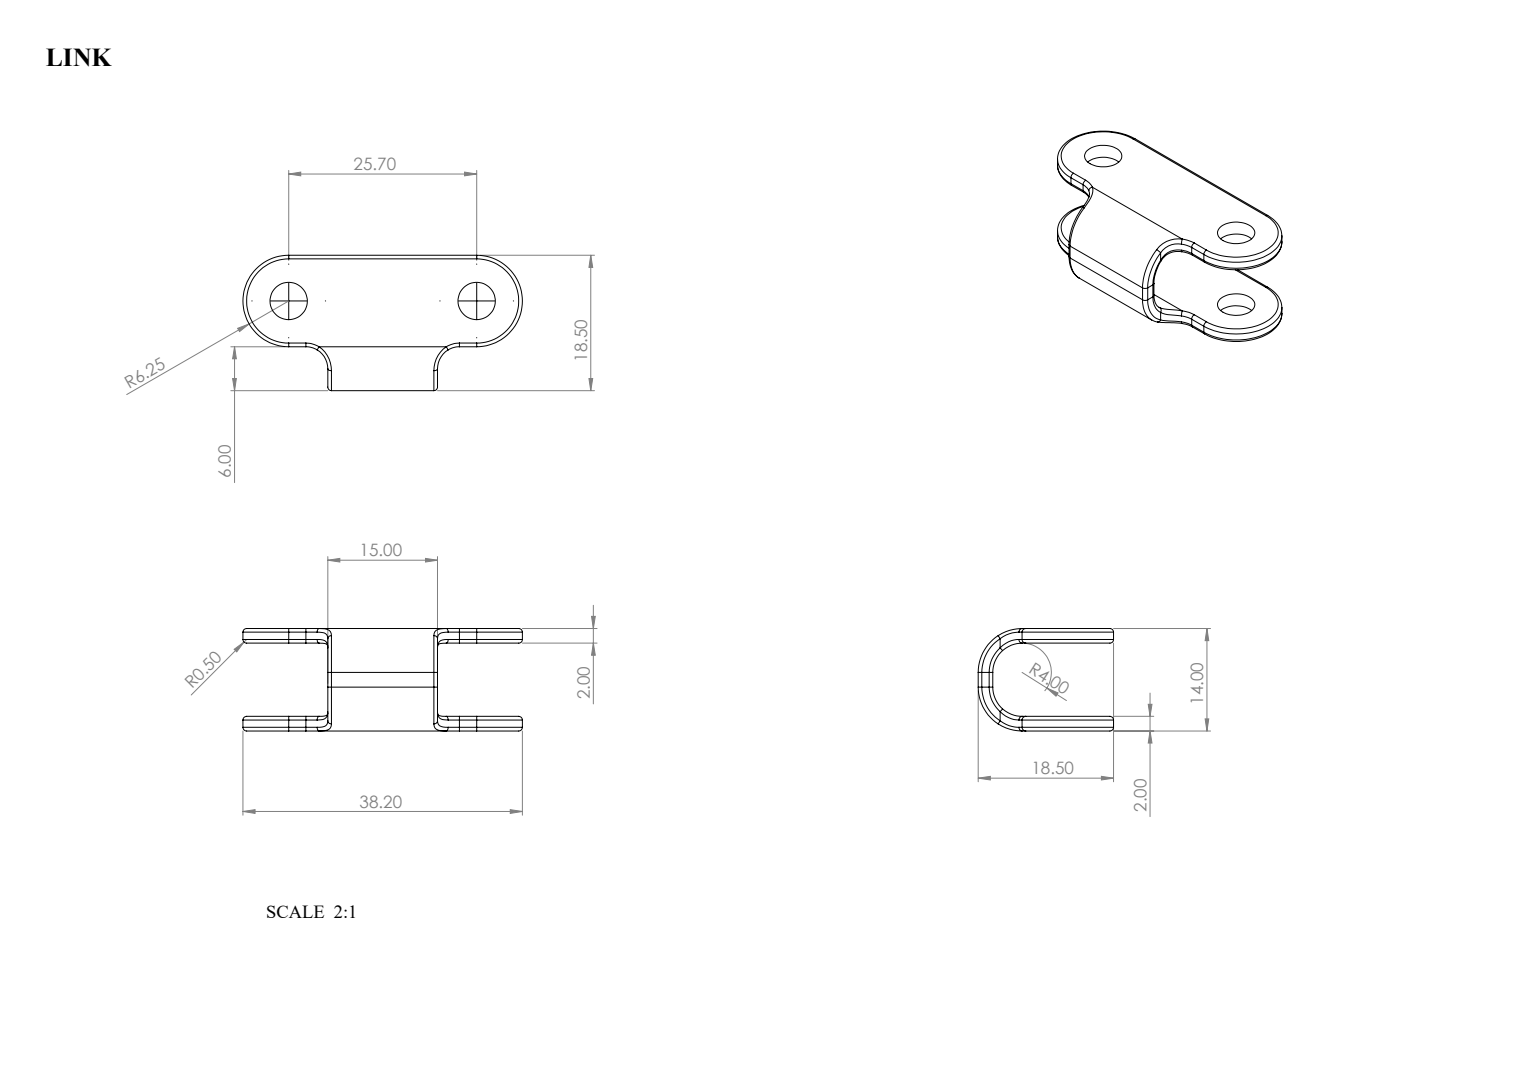
ISO-10303-21;
HEADER;
FILE_DESCRIPTION (('STEP AP214'),
    '1' );
FILE_NAME ('Link.step',
    '2026-10-06T08:09:25',
    ( '' ),
    ( '' ),
    'SwSTEP 2.0',
    'SolidWorks 2021',
    '' );
FILE_SCHEMA (( 'AUTOMOTIVE_DESIGN' ));
ENDSEC;

DATA;
#21=CARTESIAN_POINT ( 'NONE',  ( 8.498922697886333921, -1.509195795641886439, 6.997949321565420711 ) ) ;
#31=EDGE_LOOP ( 'NONE', ( #17480, #19110, #8752, #782 ) ) ;
#37=DIRECTION ( 'NONE',  ( 1.000000000000000000, 4.252453317207022018E-31, -5.551115123125818447E-17 ) ) ;
#38=ADVANCED_FACE ( 'NONE', ( #17307 ), #9922, .T. ) ;
#39=CARTESIAN_POINT ( 'NONE',  ( 7.263517083688578069, -11.72058614530574694, 7.724990489865656507 ) ) ;
#41=CARTESIAN_POINT ( 'NONE',  ( -6.999999999999978684, -10.98142396999974046, 8.916666666666724694 ) ) ;
#43=CARTESIAN_POINT ( 'NONE',  ( 7.909386411297032460, -13.36290293203342650, 7.731447622712527057 ) ) ;
#47=CARTESIAN_POINT ( 'NONE',  ( 12.84999999999997300, -1.999999999999998224, -2.550000000000000711 ) ) ;
#48=DIRECTION ( 'NONE',  ( -2.168404344971017743E-16, -1.000000000000000000, 6.982962677686261977E-15 ) ) ;
#49=DIRECTION ( 'NONE',  ( 0.000000000000000000, 0.000000000000000000, 1.000000000000000000 ) ) ;
#50=EDGE_CURVE ( 'NONE', #20148, #6938, #11790, .T. ) ;
#51=CYLINDRICAL_SURFACE ( 'NONE', #1797, 0.4999999999999995559 ) ;
#56=EDGE_LOOP ( 'NONE', ( #13558, #11700, #20158, #8031 ) ) ;
#82=CYLINDRICAL_SURFACE ( 'NONE', #15543, 0.4999999999999995559 ) ;
#89=ORIENTED_EDGE ( 'NONE', *, *, #7270, .T. ) ;
#94=CARTESIAN_POINT ( 'NONE',  ( 7.499999999999978684, 1.734723475976807094E-14, 9.249999999999980460 ) ) ;
#111=ORIENTED_EDGE ( 'NONE', *, *, #7820, .T. ) ;
#112=ORIENTED_EDGE ( 'NONE', *, *, #14818, .T. ) ;
#127=CARTESIAN_POINT ( 'NONE',  ( 7.499999999999978684, -2.645898033750298417, 9.250000000000021316 ) ) ;
#129=CARTESIAN_POINT ( 'NONE',  ( 8.697224362268009656, -1.999999999999984013, 6.249999999999998224 ) ) ;
#138=VERTEX_POINT ( 'NONE', #8274 ) ;
#149=CARTESIAN_POINT ( 'NONE',  ( 7.554637128289398262, -0.1201405311246625390, 7.453047528892632556 ) ) ;
#150=CARTESIAN_POINT ( 'NONE',  ( 8.723547172042144027, -11.98401194435536432, 6.817515300135809753 ) ) ;
#153=CARTESIAN_POINT ( 'NONE',  ( 7.000000000000006217, -11.35410196624971491, 9.250000000000008882 ) ) ;
#161=CARTESIAN_POINT ( 'NONE',  ( -12.85000000000004228, -0.5000000000000004441, -6.249999999999977796 ) ) ;
#164=DIRECTION ( 'NONE',  ( -9.121204216617949000E-31, -1.000000000000000000, 6.982962677686261977E-15 ) ) ;
#167=CARTESIAN_POINT ( 'NONE',  ( 8.204963667274160599, -0.08625821904936173401, 7.312308861538857840 ) ) ;
#193=CARTESIAN_POINT ( 'NONE',  ( -12.84999999999999964, -1.500000000000001332, 5.750000000000005329 ) ) ;
#195=VERTEX_POINT ( 'NONE', #8969 ) ;
#207=ADVANCED_FACE ( 'NONE', ( #3092, #23213, #8851 ), #10257, .T. ) ;
#208=EDGE_CURVE ( 'NONE', #21919, #22681, #22973, .T. ) ;
#211=DIRECTION ( 'NONE',  ( 1.454462294001240516E-30, 1.000000000000000000, 0.000000000000000000 ) ) ;
#213=DIRECTION ( 'NONE',  ( -2.168404344971017743E-16, -1.000000000000000000, 6.982962677686261977E-15 ) ) ;
#215=CARTESIAN_POINT ( 'NONE',  ( -8.195710046796538251, -2.011959044857179357, 6.570882465138005557 ) ) ;
#219=CARTESIAN_POINT ( 'NONE',  ( 10.49999999999999467, -14.00000000000000888, 9.250000000000063949 ) ) ;
#224=CARTESIAN_POINT ( 'NONE',  ( -10.49999999999999467, -1.500000000000001332, 5.750000000000005329 ) ) ;
#229=ORIENTED_EDGE ( 'NONE', *, *, #14979, .F. ) ;
#236=CIRCLE ( 'NONE', #19764, 2.999999999999995559 ) ;
#241=CARTESIAN_POINT ( 'NONE',  ( 8.510464245293309915, -13.49280278100692243, 6.988717072694059063 ) ) ;
#247=ORIENTED_EDGE ( 'NONE', *, *, #13683, .T. ) ;
#255=CARTESIAN_POINT ( 'NONE',  ( 7.000000000000001776, -10.98142396999974935, 8.916666666666673180 ) ) ;
#268=CARTESIAN_POINT ( 'NONE',  ( 8.565230440156003766, -1.999999999999984457, 6.320505311736929421 ) ) ;
#270=CARTESIAN_POINT ( 'NONE',  ( 8.429621201837189659, 1.585786587480479934E-14, 6.425428529984677617 ) ) ;
#280=VERTEX_POINT ( 'NONE', #12363 ) ;
#300=FACE_OUTER_BOUND ( 'NONE', #859, .T. ) ;
#303=EDGE_CURVE ( 'NONE', #3117, #17483, #12943, .T. ) ;
#313=ORIENTED_EDGE ( 'NONE', *, *, #17284, .F. ) ;
#331=DIRECTION ( 'NONE',  ( 9.121204216617949000E-31, 1.000000000000000000, -6.982962677686261977E-15 ) ) ;
#347=CARTESIAN_POINT ( 'NONE',  ( 7.500000000000007105, -5.999999999999981348, 12.24999999999998224 ) ) ;
#353=EDGE_CURVE ( 'NONE', #9717, #9721, #18241, .T. ) ;
#358=CARTESIAN_POINT ( 'NONE',  ( 7.651206356577058720, -13.16616768173521912, 8.300907142094251512 ) ) ;
#359=DIRECTION ( 'NONE',  ( 1.000000000000000000, 1.910522504832140594E-31, -5.551115123125818447E-17 ) ) ;
#392=CARTESIAN_POINT ( 'NONE',  ( 7.345446946324464932, -0.2181520686730648306, 7.860330092053914974 ) ) ;
#396=VERTEX_POINT ( 'NONE', #16803 ) ;
#398=ORIENTED_EDGE ( 'NONE', *, *, #14716, .T. ) ;
#403=CYLINDRICAL_SURFACE ( 'NONE', #5007, 2.549999999999997158 ) ;
#404=( BOUNDED_SURFACE ( )  B_SPLINE_SURFACE ( 3, 2, ( 
 ( #12933, #11388, #19885 ),
 ( #2337, #3867, #21995 ),
 ( #16676, #20341, #11045 ),
 ( #16449, #5881, #465 ),
 ( #1987, #21769, #358 ),
 ( #5654, #9411, #3752 ),
 ( #13050, #20237, #11166 ),
 ( #587, #6112, #14923 ),
 ( #7871, #22109, #18578 ),
 ( #6001, #16555, #7527 ),
 ( #2228, #15035, #10918 ),
 ( #9177, #16338, #241 ),
 ( #7412, #20827, #6346 ),
 ( #4690, #13397, #13518 ) ),
 .UNSPECIFIED., .F., .F., .F. ) 
 B_SPLINE_SURFACE_WITH_KNOTS ( ( 4, 2, 2, 2, 2, 2, 4 ),
 ( 3, 3 ),
 ( 0.000000000000000000, 0.0009385527998839217345, 0.001407829199825882602, 0.001877105599767843469, 0.002346381999709804336, 0.002815658399651765204, 0.003754211199535686938 ),
 ( 0.000000000000000000, 1.000000000000000000 ),
 .UNSPECIFIED. ) 
 GEOMETRIC_REPRESENTATION_ITEM ( )  RATIONAL_B_SPLINE_SURFACE ( (
 ( 1.000000000000000000, 0.7071067811865469066, 1.000000000000000000),
 ( 1.000000000000000000, 0.7217349950160889538, 1.000000000000000000),
 ( 1.000000000000000000, 0.7325631490734629825, 1.000000000000000000),
 ( 1.000000000000000000, 0.7426392126584471232, 1.000000000000000000),
 ( 1.000000000000000000, 0.7449451721693458595, 1.000000000000000000),
 ( 1.000000000000000000, 0.7474053618999159099, 1.000000000000000000),
 ( 1.000000000000000000, 0.7475947887410098192, 1.000000000000000000),
 ( 1.000000000000000000, 0.7461109904165789120, 1.000000000000000000),
 ( 1.000000000000000000, 0.7444113185333037785, 1.000000000000000000),
 ( 1.000000000000000000, 0.7395217850810181792, 1.000000000000000000),
 ( 1.000000000000000000, 0.7363545993504778675, 1.000000000000000000),
 ( 1.000000000000000000, 0.7253814056383908193, 1.000000000000000000),
 ( 1.000000000000000000, 0.7159765610437973660, 1.000000000000000000),
 ( 1.000000000000000000, 0.7071067811865494601, 1.000000000000000000) ) ) 
 REPRESENTATION_ITEM ( '' )  SURFACE ( )  );
#406=ORIENTED_EDGE ( 'NONE', *, *, #6745, .T. ) ;
#413=FACE_OUTER_BOUND ( 'NONE', #17566, .T. ) ;
#420=ORIENTED_EDGE ( 'NONE', *, *, #15029, .F. ) ;
#422=ORIENTED_EDGE ( 'NONE', *, *, #14825, .T. ) ;
#431=CARTESIAN_POINT ( 'NONE',  ( -12.85000000000001386, -14.00000000000005329, 2.550000000000052669 ) ) ;
#453=CARTESIAN_POINT ( 'NONE',  ( -12.84999999999999964, -0.5000000000000038858, 5.750000000000018652 ) ) ;
#458=AXIS2_PLACEMENT_3D ( 'NONE', #20608, #18832, #22132 ) ;
#463=AXIS2_PLACEMENT_3D ( 'NONE', #5270, #12430, #19613 ) ;
#465=CARTESIAN_POINT ( 'NONE',  ( 7.613388670473287156, -13.11165441297993084, 8.423574099071744925 ) ) ;
#469=PRESENTATION_STYLE_ASSIGNMENT (( #14587 ) ) ;
#476=CIRCLE ( 'NONE', #11356, 0.4999999999999998335 ) ;
#479=AXIS2_PLACEMENT_3D ( 'NONE', #21483, #5360, #14060 ) ;
#501=DIRECTION ( 'NONE',  ( 1.454462294001240516E-30, 1.000000000000000000, 0.000000000000000000 ) ) ;
#508=CARTESIAN_POINT ( 'NONE',  ( 7.000000000000009770, -0.9711575687493200215, 9.522727272727296466 ) ) ;
#523=CIRCLE ( 'NONE', #891, 4.000000000000000000 ) ;
#525=AXIS2_PLACEMENT_3D ( 'NONE', #3093, #22741, #3329 ) ;
#526=DIRECTION ( 'NONE',  ( -1.000000000000000000, -6.224605580259554159E-31, 2.887593071917436153E-31 ) ) ;
#532=DIRECTION ( 'NONE',  ( -1.000000000000000000, 2.312964634635739999E-16, -1.302601544865244959E-30 ) ) ;
#538=VECTOR ( 'NONE', #11676, 1000.000000000000000 ) ;
#540=ORIENTED_EDGE ( 'NONE', *, *, #22390, .T. ) ;
#562=CARTESIAN_POINT ( 'NONE',  ( -8.422565759993579704, -12.00000000000004441, 6.396710472006764903 ) ) ;
#563=CARTESIAN_POINT ( 'NONE',  ( -7.604097569491910846, -13.58924811263090504, 8.440516644273101221 ) ) ;
#579=CARTESIAN_POINT ( 'NONE',  ( -8.954763739086851970, -12.50000000000002132, 6.678571428571506097 ) ) ;
#587=CARTESIAN_POINT ( 'NONE',  ( 7.490313984279763027, -13.85571552873294365, 7.566633644154762806 ) ) ;
#597=EDGE_CURVE ( 'NONE', #11755, #7710, #15633, .T. ) ;
#605=ORIENTED_EDGE ( 'NONE', *, *, #6240, .F. ) ;
#617=EDGE_CURVE ( 'NONE', #18641, #4863, #6775, .T. ) ;
#618=FACE_OUTER_BOUND ( 'NONE', #20038, .T. ) ;
#635=VERTEX_POINT ( 'NONE', #18338 ) ;
#639=CYLINDRICAL_SURFACE ( 'NONE', #14898, 2.549999999999997158 ) ;
#642=CARTESIAN_POINT ( 'NONE',  ( 8.954763739086866181, -13.50000000000002309, 6.678571428571478563 ) ) ;
#706=CARTESIAN_POINT ( 'NONE',  ( 8.160037397871480636, -13.99120688549555425, 6.662331851012024408 ) ) ;
#711=FILL_AREA_STYLE_COLOUR ( '', #14886 ) ;
#723=ADVANCED_FACE ( 'NONE', ( #1644 ), #6821, .F. ) ;
#734=DIRECTION ( 'NONE',  ( -2.168404344970994323E-16, 1.000000000000000000, -1.577721810442023611E-30 ) ) ;
#742=ORIENTED_EDGE ( 'NONE', *, *, #2797, .T. ) ;
#760=CARTESIAN_POINT ( 'NONE',  ( -7.521298409251860662, -2.242072331701493670, 8.817899680514866390 ) ) ;
#765=CARTESIAN_POINT ( 'NONE',  ( -12.84999999999999964, -2.000000000000001776, 0.000000000000000000 ) ) ;
#780=ORIENTED_EDGE ( 'NONE', *, *, #14197, .F. ) ;
#782=ORIENTED_EDGE ( 'NONE', *, *, #10105, .F. ) ;
#791=AXIS2_PLACEMENT_3D ( 'NONE', #11762, #9654, #13189 ) ;
#793=CARTESIAN_POINT ( 'NONE',  ( -7.568091547083489523, -11.30436690654930310, 8.516664522246358615 ) ) ;
#794=CARTESIAN_POINT ( 'NONE',  ( -7.856071383949657871, -13.95231939088843021, 7.015054140272262373 ) ) ;
#799=CARTESIAN_POINT ( 'NONE',  ( -12.84999999999999964, -1.500000000000001332, 5.750000000000005329 ) ) ;
#807=CARTESIAN_POINT ( 'NONE',  ( -12.84999999999999964, -1.500000000000001332, 0.000000000000000000 ) ) ;
#809=B_SPLINE_CURVE_WITH_KNOTS ( 'NONE', 3,
 ( #13972, #21165, #12198, #1513, #14095, #21281, #3840, #18320, #5628, #11357, #21972, #19968, #19857, #9491, #4079, #7847 ),
 .UNSPECIFIED., .F., .F.,
 ( 4, 2, 2, 2, 2, 2, 2, 4 ),
 ( 2.168404344970985372E-18, 0.0008458391445145506393, 0.001268758716771827043, 0.001691678289029103664, 0.002114597861286380068, 0.002537517433543656688, 0.002960437005800932875, 0.003383356578058209496 ),
 .UNSPECIFIED. ) ;
#810=DIRECTION ( 'NONE',  ( 1.000000000000000000, 3.081487911019581306E-31, -5.551115123125761132E-17 ) ) ;
#828=ORIENTED_EDGE ( 'NONE', *, *, #7076, .T. ) ;
#840=DIRECTION ( 'NONE',  ( 1.000000000000000000, -2.168404344971017743E-16, 1.203141491611691375E-30 ) ) ;
#848=DIRECTION ( 'NONE',  ( 2.168404344971008868E-16, 1.000000000000000000, 0.000000000000000000 ) ) ;
#859=EDGE_LOOP ( 'NONE', ( #22643, #18058, #20307, #6787 ) ) ;
#877=EDGE_CURVE ( 'NONE', #9710, #18942, #14680, .T. ) ;
#891=AXIS2_PLACEMENT_3D ( 'NONE', #18596, #17276, #8120 ) ;
#898=ADVANCED_FACE ( 'NONE', ( #12924 ), #16547, .T. ) ;
#911=CARTESIAN_POINT ( 'NONE',  ( -7.024848138041019041, -11.34038014973646646, 8.468562630484528952 ) ) ;
#915=EDGE_CURVE ( 'NONE', #19164, #20509, #11154, .T. ) ;
#922=CARTESIAN_POINT ( 'NONE',  ( 7.000000000000006217, -5.999999999999981348, 6.250000000000005329 ) ) ;
#923=ORIENTED_EDGE ( 'NONE', *, *, #303, .F. ) ;
#925=TOROIDAL_SURFACE ( 'NONE', #3908, 3.500000000000000000, 0.5000000000000000000 ) ;
#930=TOROIDAL_SURFACE ( 'NONE', #11052, 5.750000000000000000, 0.5000000000000000000 ) ;
#938=LINE ( 'NONE', #22804, #4058 ) ;
#940=DIRECTION ( 'NONE',  ( -9.121204216617949000E-31, -1.000000000000000000, 6.982962677686261977E-15 ) ) ;
#948=DIRECTION ( 'NONE',  ( -0.8571428571428582055, -3.574076823648845814E-15, -0.5150787536377109399 ) ) ;
#952=ORIENTED_EDGE ( 'NONE', *, *, #22611, .T. ) ;
#958=CARTESIAN_POINT ( 'NONE',  ( -12.85000000000001386, -14.00000000000007105, 5.551115123125782702E-14 ) ) ;
#967=CARTESIAN_POINT ( 'NONE',  ( 10.49999999999999467, -12.50000000000000711, 9.250000000000063949 ) ) ;
#975=ORIENTED_EDGE ( 'NONE', *, *, #6535, .T. ) ;
#978=ORIENTED_EDGE ( 'NONE', *, *, #8806, .F. ) ;
#1022=CARTESIAN_POINT ( 'NONE',  ( -7.854293383767468661, -11.68772904158800507, 7.820081954007019220 ) ) ;
#1023=CARTESIAN_POINT ( 'NONE',  ( -8.204963667274178363, -13.91374178095054504, 7.312308861539002613 ) ) ;
#1028=CARTESIAN_POINT ( 'NONE',  ( 6.999999999999992006, -8.000000000000051514, 6.249999999999977796 ) ) ;
#1042=EDGE_CURVE ( 'NONE', #11093, #19516, #20692, .T. ) ;
#1044=ORIENTED_EDGE ( 'NONE', *, *, #18492, .T. ) ;
#1050=ADVANCED_FACE ( 'NONE', ( #4683 ), #7758, .T. ) ;
#1056=VECTOR ( 'NONE', #20372, 1000.000000000000000 ) ;
#1074=CIRCLE ( 'NONE', #6325, 5.500000000000000000 ) ;
#1078=ORIENTED_EDGE ( 'NONE', *, *, #19074, .F. ) ;
#1081=CARTESIAN_POINT ( 'NONE',  ( 7.499999999999978684, -8.000000000000051514, 6.249999999999977796 ) ) ;
#1085=PLANE ( 'NONE',  #6581 ) ;
#1089=DIRECTION ( 'NONE',  ( 0.000000000000000000, 0.000000000000000000, 1.000000000000000000 ) ) ;
#1105=CARTESIAN_POINT ( 'NONE',  ( -6.999999999999992006, -5.999999999999987566, 6.250000000000005329 ) ) ;
#1112=CARTESIAN_POINT ( 'NONE',  ( -8.719386969281453403, -1.499999991380633446, 6.820015264002448951 ) ) ;
#1113=CARTESIAN_POINT ( 'NONE',  ( -12.85000000000005649, -13.50000000000011191, -6.249999999999921840 ) ) ;
#1115=CARTESIAN_POINT ( 'NONE',  ( 10.49999999999996803, -0.5000000000000004441, 5.750000000000032863 ) ) ;
#1143=CARTESIAN_POINT ( 'NONE',  ( -7.756475484083226846, -13.93440482874970066, 7.145789564688727502 ) ) ;
#1144=DIRECTION ( 'NONE',  ( -9.121204216617949000E-31, -1.000000000000000000, 6.982962677686276966E-15 ) ) ;
#1147=PLANE ( 'NONE',  #16386 ) ;
#1155=VERTEX_POINT ( 'NONE', #1726 ) ;
#1161=AXIS2_PLACEMENT_3D ( 'NONE', #5449, #12957, #8972 ) ;
#1168=CARTESIAN_POINT ( 'NONE',  ( -7.742458795615052125, -0.7399311281351333980, 8.061568688625936119 ) ) ;
#1171=LINE ( 'NONE', #18813, #22070 ) ;
#1174=CARTESIAN_POINT ( 'NONE',  ( -8.697224362267968800, -13.50000000000004263, 6.250000000000033751 ) ) ;
#1175=AXIS2_PLACEMENT_3D ( 'NONE', #17283, #13886, #10583 ) ;
#1177=ADVANCED_FACE ( 'NONE', ( #1503 ), #3393, .T. ) ;
#1187=ORIENTED_EDGE ( 'NONE', *, *, #22325, .T. ) ;
#1192=DIRECTION ( 'NONE',  ( -1.000000000000000000, -2.168404344971017743E-16, 1.780660105995169760E-30 ) ) ;
#1201=VERTEX_POINT ( 'NONE', #15951 ) ;
#1206=VERTEX_POINT ( 'NONE', #1388 ) ;
#1215=DIRECTION ( 'NONE',  ( 1.734723475976813750E-16, 1.000000000000000000, -3.469446951953607484E-15 ) ) ;
#1219=CARTESIAN_POINT ( 'NONE',  ( -7.028413389564923897, -0.6300521812368727881, 8.946655872545999699 ) ) ;
#1230=CARTESIAN_POINT ( 'NONE',  ( -7.764145988665059228, -12.22513543353773002, 8.011880279048888553 ) ) ;
#1252=DIRECTION ( 'NONE',  ( -4.019602852144232182E-47, -6.982962677686261977E-15, -1.000000000000000000 ) ) ;
#1258=DIRECTION ( 'NONE',  ( -1.000000000000000000, 2.168404344971005170E-16, -1.203141491611682442E-30 ) ) ;
#1264=PRESENTATION_STYLE_ASSIGNMENT (( #18908 ) ) ;
#1266=CARTESIAN_POINT ( 'NONE',  ( -7.500000000000007105, -11.35410196624970780, 9.250000000000035527 ) ) ;
#1273=DIRECTION ( 'NONE',  ( 0.000000000000000000, 0.000000000000000000, 1.000000000000000000 ) ) ;
#1278=CIRCLE ( 'NONE', #11789, 3.499999999999996003 ) ;
#1282=CARTESIAN_POINT ( 'NONE',  ( -7.500000000000007105, 1.387778780781445676E-14, 6.249999999999992006 ) ) ;
#1285=CARTESIAN_POINT ( 'NONE',  ( -7.490313984279710624, -0.1442844712670970087, 7.566633644154755700 ) ) ;
#1295=ORIENTED_EDGE ( 'NONE', *, *, #18492, .F. ) ;
#1316=CARTESIAN_POINT ( 'NONE',  ( -7.499999999999992895, -5.999999999999987566, 6.249999999999992006 ) ) ;
#1334=ADVANCED_FACE ( 'NONE', ( #20519 ), #639, .F. ) ;
#1336=CARTESIAN_POINT ( 'NONE',  ( 10.50000000000000888, -0.5000000000000004441, 9.250000000000008882 ) ) ;
#1337=CARTESIAN_POINT ( 'NONE',  ( -7.554637128289355630, -0.1201405311246572377, 7.453047528892588147 ) ) ;
#1342=AXIS2_PLACEMENT_3D ( 'NONE', #958, #10123, #18822 ) ;
#1344=CARTESIAN_POINT ( 'NONE',  ( -8.697224362268011433, -0.4999999999999970024, 6.250000000000033751 ) ) ;
#1351=ORIENTED_EDGE ( 'NONE', *, *, #2302, .T. ) ;
#1362=DIRECTION ( 'NONE',  ( 0.000000000000000000, 3.469446951953619316E-15, 1.000000000000000000 ) ) ;
#1377=CARTESIAN_POINT ( 'NONE',  ( -8.832214555408084422, -1.499999999999987343, 6.752214322824768189 ) ) ;
#1388=CARTESIAN_POINT ( 'NONE',  ( -10.49999999999996803, -6.938893903907228378E-15, 5.749999999999976907 ) ) ;
#1392=EDGE_CURVE ( 'NONE', #13556, #12774, #13038, .T. ) ;
#1398=DIRECTION ( 'NONE',  ( 9.121204216617949000E-31, 1.000000000000000000, -6.982962677686261977E-15 ) ) ;
#1400=CARTESIAN_POINT ( 'NONE',  ( -12.84999999999999964, 0.000000000000000000, 0.000000000000000000 ) ) ;
#1405=VECTOR ( 'NONE', #13055, 1000.000000000000000 ) ;
#1420=AXIS2_PLACEMENT_3D ( 'NONE', #19154, #10205, #5034 ) ;
#1441=AXIS2_PLACEMENT_3D ( 'NONE', #19500, #6925, #1618 ) ;
#1443=CARTESIAN_POINT ( 'NONE',  ( 7.499999999999978684, -12.60977222864647196, 9.250000000000049738 ) ) ;
#1446=CARTESIAN_POINT ( 'NONE',  ( 7.000000000000006217, -5.999999999999981348, 10.24999999999998224 ) ) ;
#1447=AXIS2_PLACEMENT_3D ( 'NONE', #6198, #17344, #1252 ) ;
#1463=ORIENTED_EDGE ( 'NONE', *, *, #14109, .T. ) ;
#1466=EDGE_CURVE ( 'NONE', #16593, #10367, #6244, .T. ) ;
#1468=CARTESIAN_POINT ( 'NONE',  ( -12.84999999999999964, -12.50000000000006928, 6.938893903907228378E-14 ) ) ;
#1498=ORIENTED_EDGE ( 'NONE', *, *, #3492, .T. ) ;
#1499=CARTESIAN_POINT ( 'NONE',  ( -7.000000000000020428, -5.999999999999981348, 10.74999999999996803 ) ) ;
#1501=EDGE_CURVE ( 'NONE', #20416, #635, #236, .T. ) ;
#1503=FACE_OUTER_BOUND ( 'NONE', #18223, .T. ) ;
#1507=CYLINDRICAL_SURFACE ( 'NONE', #1441, 2.549999999999997158 ) ;
#1509=CARTESIAN_POINT ( 'NONE',  ( -7.132286784435581950, -0.4236497315829815813, 8.470912490188249322 ) ) ;
#1513=CARTESIAN_POINT ( 'NONE',  ( 7.595478965369728108, -2.023942297479887742, 8.489833260407438686 ) ) ;
#1516=DIRECTION ( 'NONE',  ( -1.927470528863118556E-16, 1.000000000000000000, 0.000000000000000000 ) ) ;
#1517=DIRECTION ( 'NONE',  ( 2.168404344971017743E-16, 1.000000000000000000, -6.982962677686261977E-15 ) ) ;
#1531=ORIENTED_EDGE ( 'NONE', *, *, #16518, .F. ) ;
#1535=CARTESIAN_POINT ( 'NONE',  ( -7.473326079327797800, -13.84852298796451464, 7.598194856234270489 ) ) ;
#1540=LINE ( 'NONE', #8714, #5955 ) ;
#1546=VERTEX_POINT ( 'NONE', #12368 ) ;
#1548=VECTOR ( 'NONE', #20577, 1000.000000000000000 ) ;
#1563=ADVANCED_FACE ( 'NONE', ( #19908 ), #16365, .T. ) ;
#1570=ORIENTED_EDGE ( 'NONE', *, *, #9831, .F. ) ;
#1574=EDGE_LOOP ( 'NONE', ( #5344, #16025, #6543, #19081 ) ) ;
#1584=DIRECTION ( 'NONE',  ( 0.000000000000000000, 0.000000000000000000, -1.000000000000000000 ) ) ;
#1585=ADVANCED_FACE ( 'NONE', ( #14263 ), #17498, .T. ) ;
#1593=CIRCLE ( 'NONE', #6099, 6.249999999999992006 ) ;
#1598=CARTESIAN_POINT ( 'NONE',  ( 12.84999999999997300, -0.5000000000000004441, -6.249999999999963585 ) ) ;
#1601=EDGE_CURVE ( 'NONE', #8927, #10359, #20790, .T. ) ;
#1606=CIRCLE ( 'NONE', #8742, 6.249999999999992006 ) ;
#1618=DIRECTION ( 'NONE',  ( 0.000000000000000000, 6.802837160693368935E-15, 1.000000000000000000 ) ) ;
#1619=DIRECTION ( 'NONE',  ( 0.000000000000000000, 0.000000000000000000, 1.000000000000000000 ) ) ;
#1636=EDGE_CURVE ( 'NONE', #7030, #18641, #5864, .T. ) ;
#1644=FACE_OUTER_BOUND ( 'NONE', #14527, .T. ) ;
#1657=CARTESIAN_POINT ( 'NONE',  ( -12.85000000000001386, -14.00000000000007105, 5.551115123125782702E-14 ) ) ;
#1662=DIRECTION ( 'NONE',  ( 0.000000000000000000, 0.000000000000000000, 1.000000000000000000 ) ) ;
#1686=CARTESIAN_POINT ( 'NONE',  ( 12.84999999999997300, -12.50000000000006928, 5.551115123125782702E-14 ) ) ;
#1690=DIRECTION ( 'NONE',  ( 9.121204216617949000E-31, 1.000000000000000000, -6.982962677686261977E-15 ) ) ;
#1708=CARTESIAN_POINT ( 'NONE',  ( -12.84999999999999964, -6.938893903907228378E-15, 5.749999999999991118 ) ) ;
#1713=CARTESIAN_POINT ( 'NONE',  ( 7.500000000000007105, -5.999999999999981348, 12.24999999999998224 ) ) ;
#1715=CARTESIAN_POINT ( 'NONE',  ( -7.500000000000007105, -2.645898033750305522, 9.250000000000035527 ) ) ;
#1726=CARTESIAN_POINT ( 'NONE',  ( -10.49999999999999467, -2.000000000000001776, 5.750000000000005329 ) ) ;
#1731=DIRECTION ( 'NONE',  ( 2.168404344970994323E-16, -1.000000000000000000, 1.577721810442023611E-30 ) ) ;
#1753=ADVANCED_FACE ( 'NONE', ( #18476 ), #20244, .T. ) ;
#1754=EDGE_LOOP ( 'NONE', ( #12623, #1498, #12008, #18274 ) ) ;
#1760=CARTESIAN_POINT ( 'NONE',  ( -8.160037397871475306, -13.99120688549555602, 6.662331851011996875 ) ) ;
#1762=CARTESIAN_POINT ( 'NONE',  ( 8.954763739086869734, -1.499999999999984013, 6.678571428571429713 ) ) ;
#1778=ORIENTED_EDGE ( 'NONE', *, *, #3061, .F. ) ;
#1784=CARTESIAN_POINT ( 'NONE',  ( -7.268749084027625429, -11.74104661578623521, 7.689023314178108137 ) ) ;
#1788=CARTESIAN_POINT ( 'NONE',  ( 8.718376657154827569, -13.50000000000004086, 6.820622386032026974 ) ) ;
#1789=AXIS2_PLACEMENT_3D ( 'NONE', #3022, #2791, #22555 ) ;
#1797=AXIS2_PLACEMENT_3D ( 'NONE', #12494, #3572, #12734 ) ;
#1800=CARTESIAN_POINT ( 'NONE',  ( 8.725359747074517003, -0.4999999928004930649, 6.816426071237541073 ) ) ;
#1809=ORIENTED_EDGE ( 'NONE', *, *, #8067, .T. ) ;
#1826=CARTESIAN_POINT ( 'NONE',  ( -8.715898959466867879, -1.502431622389268417, 6.833978265953976283 ) ) ;
#1840=VECTOR ( 'NONE', #12414, 1000.000000000000000 ) ;
#1843=CARTESIAN_POINT ( 'NONE',  ( 8.832214555408096857, -12.50000000000003375, 6.752214322824835691 ) ) ;
#1846=CARTESIAN_POINT ( 'NONE',  ( 10.50000000000000888, -1.500000000000001332, 5.750000000000005329 ) ) ;
#1856=SHAPE_REPRESENTATION ( 'Link', ( #22115 ), #3350 ) ;
#1877=ORIENTED_EDGE ( 'NONE', *, *, #8108, .T. ) ;
#1888=CARTESIAN_POINT ( 'NONE',  ( 7.972478112619588941, -12.36350260656811528, 7.628219499134369919 ) ) ;
#1902=FACE_OUTER_BOUND ( 'NONE', #22361, .T. ) ;
#1931=CARTESIAN_POINT ( 'NONE',  ( 12.84999999999997300, -14.00000000000005329, 2.550000000000052669 ) ) ;
#1937=ORIENTED_EDGE ( 'NONE', *, *, #9948, .T. ) ;
#1951=PLANE ( 'NONE',  #19958 ) ;
#1958=VECTOR ( 'NONE', #17366, 1000.000000000000000 ) ;
#1961=TOROIDAL_SURFACE ( 'NONE', #15481, 3.500000000000000000, 0.5000000000000000000 ) ;
#1978=CARTESIAN_POINT ( 'NONE',  ( 8.565230440156009095, -12.00000000000005151, 6.320505311736963172 ) ) ;
#1986=CARTESIAN_POINT ( 'NONE',  ( 7.735962016526152674, -13.93008758169059469, 7.174192622767042948 ) ) ;
#1987=CARTESIAN_POINT ( 'NONE',  ( 7.176407415342080043, -13.63581929081302668, 8.314790908397570846 ) ) ;
#2007=CARTESIAN_POINT ( 'NONE',  ( 8.165409815605739752, -11.99182595524110084, 6.581206704444357847 ) ) ;
#2010=CARTESIAN_POINT ( 'NONE',  ( -6.999999999999976907, -11.18103031733298280, 8.693499985977949152 ) ) ;
#2013=LINE ( 'NONE', #7550, #15143 ) ;
#2021=DIRECTION ( 'NONE',  ( -1.000000000000000000, 0.000000000000000000, 0.000000000000000000 ) ) ;
#2026=CARTESIAN_POINT ( 'NONE',  ( 8.721922330811608504, -0.01237189218583836445, 6.818491697976307719 ) ) ;
#2036=EDGE_LOOP ( 'NONE', ( #4334, #5262, #8876, #17329 ) ) ;
#2038=CARTESIAN_POINT ( 'NONE',  ( 12.84999999999995879, -12.50000000000011191, -5.749999999999907629 ) ) ;
#2051=DIRECTION ( 'NONE',  ( 1.000000000000000000, 2.168404344971017743E-16, -1.780660105995169760E-30 ) ) ;
#2064=ADVANCED_FACE ( 'NONE', ( #14470 ), #17762, .T. ) ;
#2077=EDGE_CURVE ( 'NONE', #8641, #18911, #11561, .T. ) ;
#2080=DIRECTION ( 'NONE',  ( 0.000000000000000000, -6.938893903907237844E-15, -1.000000000000000000 ) ) ;
#2096=CARTESIAN_POINT ( 'NONE',  ( 12.84999999999999964, -2.000000000000005329, -5.749999999999991118 ) ) ;
#2116=VERTEX_POINT ( 'NONE', #2452 ) ;
#2121=CARTESIAN_POINT ( 'NONE',  ( 7.551224464536113956, -11.87866898603340537, 7.234820221745447810 ) ) ;
#2128=AXIS2_PLACEMENT_3D ( 'NONE', #16901, #17251, #6337 ) ;
#2135=CARTESIAN_POINT ( 'NONE',  ( 8.195710046796573778, -2.011959044857176249, 6.570882465138042861 ) ) ;
#2138=CARTESIAN_POINT ( 'NONE',  ( 8.954763739086839536, 1.073360150760649390E-14, 6.678571428571445701 ) ) ;
#2150=DIRECTION ( 'NONE',  ( 0.000000000000000000, 0.000000000000000000, 1.000000000000000000 ) ) ;
#2152=ORIENTED_EDGE ( 'NONE', *, *, #4473, .F. ) ;
#2156=AXIS2_PLACEMENT_3D ( 'NONE', #18344, #16552, #7636 ) ;
#2159=CARTESIAN_POINT ( 'NONE',  ( -7.638377885296698366, -1.936221580213996374, 8.340398698103385300 ) ) ;
#2196=EDGE_CURVE ( 'NONE', #5465, #195, #14566, .T. ) ;
#2198=CIRCLE ( 'NONE', #9730, 0.4999999999999995559 ) ;
#2202=LINE ( 'NONE', #5861, #3888 ) ;
#2203=CARTESIAN_POINT ( 'NONE',  ( -12.84999999999998721, -12.50000000000002842, 5.750000000000060396 ) ) ;
#2208=( GEOMETRIC_REPRESENTATION_CONTEXT ( 3 ) GLOBAL_UNCERTAINTY_ASSIGNED_CONTEXT ( ( #9789 ) ) GLOBAL_UNIT_ASSIGNED_CONTEXT ( ( #15597, #17476, #8547 ) ) REPRESENTATION_CONTEXT ( 'NONE', 'WORKASPACE' ) );
#2212=EDGE_CURVE ( 'NONE', #10962, #22329, #19836, .T. ) ;
#2219=CARTESIAN_POINT ( 'NONE',  ( 8.195710046796559567, -11.98804095514285173, 6.570882465138090822 ) ) ;
#2221=LINE ( 'NONE', #15463, #7149 ) ;
#2228=CARTESIAN_POINT ( 'NONE',  ( 7.856071383949645437, -13.95231939088842488, 7.015054140272347638 ) ) ;
#2238=VERTEX_POINT ( 'NONE', #15258 ) ;
#2246=CARTESIAN_POINT ( 'NONE',  ( 7.971461718369340588, -11.76779483280627048, 7.625732677302466733 ) ) ;
#2260=CARTESIAN_POINT ( 'NONE',  ( 7.748687480237993697, -0.2688970177183283572, 8.040801957829158297 ) ) ;
#2275=DIRECTION ( 'NONE',  ( -1.454462294001240516E-30, -1.000000000000000000, -0.000000000000000000 ) ) ;
#2276=ORIENTED_EDGE ( 'NONE', *, *, #9187, .T. ) ;
#2289=ORIENTED_EDGE ( 'NONE', *, *, #5634, .T. ) ;
#2301=FACE_BOUND ( 'NONE', #21032, .T. ) ;
#2302=EDGE_CURVE ( 'NONE', #5891, #2238, #938, .T. ) ;
#2306=CARTESIAN_POINT ( 'NONE',  ( -8.165409815605745081, -11.99182595524112571, 6.581206704444157118 ) ) ;
#2307=CARTESIAN_POINT ( 'NONE',  ( -7.490952241692505176, -13.34551170378494689, 8.992386117842826820 ) ) ;
#2312=FACE_OUTER_BOUND ( 'NONE', #10227, .T. ) ;
#2323=ADVANCED_FACE ( 'NONE', ( #10556 ), #1507, .F. ) ;
#2337=CARTESIAN_POINT ( 'NONE',  ( 6.999999995237020656, -13.21736471697188797, 9.233045673661203878 ) ) ;
#2360=CARTESIAN_POINT ( 'NONE',  ( -12.85000000000002807, -13.50000000000003020, 6.250000000000033751 ) ) ;
#2363=FACE_OUTER_BOUND ( 'NONE', #13769, .T. ) ;
#2364=AXIS2_PLACEMENT_3D ( 'NONE', #14718, #13078, #2598 ) ;
#2374=FACE_OUTER_BOUND ( 'NONE', #5466, .T. ) ;
#2398=CARTESIAN_POINT ( 'NONE',  ( 7.499999999999978684, -12.60977222864647196, 9.250000000000049738 ) ) ;
#2427=CARTESIAN_POINT ( 'NONE',  ( -8.438463404362648745, -2.001835333048896715, 6.398712851742144103 ) ) ;
#2430=LINE ( 'NONE', #20210, #22685 ) ;
#2438=ORIENTED_EDGE ( 'NONE', *, *, #6240, .T. ) ;
#2442=ORIENTED_EDGE ( 'NONE', *, *, #22740, .F. ) ;
#2452=CARTESIAN_POINT ( 'NONE',  ( -12.84999999999999964, 0.000000000000000000, -2.550000000000000711 ) ) ;
#2455=CARTESIAN_POINT ( 'NONE',  ( -7.000000000000006217, -8.000000000000017764, 10.24999999999999467 ) ) ;
#2465=ORIENTED_EDGE ( 'NONE', *, *, #5784, .T. ) ;
#2472=VECTOR ( 'NONE', #9416, 1000.000000000000000 ) ;
#2485=CARTESIAN_POINT ( 'NONE',  ( 7.499999999999965361, -14.00000000000003020, 9.250000000000021316 ) ) ;
#2491=ORIENTED_EDGE ( 'NONE', *, *, #14431, .F. ) ;
#2494=ADVANCED_FACE ( 'NONE', ( #13247 ), #6075, .F. ) ;
#2499=ORIENTED_EDGE ( 'NONE', *, *, #15948, .F. ) ;
#2511=FACE_OUTER_BOUND ( 'NONE', #12858, .T. ) ;
#2518=ORIENTED_EDGE ( 'NONE', *, *, #1466, .T. ) ;
#2530=EDGE_LOOP ( 'NONE', ( #21268, #3944, #20296, #7541 ) ) ;
#2532=CARTESIAN_POINT ( 'NONE',  ( -7.499999999999992895, -8.000000000000003553, 11.74999999999999645 ) ) ;
#2540=DIRECTION ( 'NONE',  ( -0.5150787536377141596, 0.000000000000000000, -0.8571428571428563181 ) ) ;
#2542=CARTESIAN_POINT ( 'NONE',  ( -7.490313984279750592, -13.85571552873294188, 7.566633644154753924 ) ) ;
#2554=ORIENTED_EDGE ( 'NONE', *, *, #22201, .F. ) ;
#2558=FACE_OUTER_BOUND ( 'NONE', #8206, .T. ) ;
#2559=DIRECTION ( 'NONE',  ( -2.168404344971017743E-16, 1.000000000000000000, 7.722382221513089478E-47 ) ) ;
#2566=CIRCLE ( 'NONE', #7831, 0.4999999999999993894 ) ;
#2571=ADVANCED_FACE ( 'NONE', ( #7722 ), #7604, .F. ) ;
#2585=ORIENTED_EDGE ( 'NONE', *, *, #2797, .F. ) ;
#2597=AXIS2_PLACEMENT_3D ( 'NONE', #11130, #14661, #20203 ) ;
#2598=DIRECTION ( 'NONE',  ( 1.000000000000000000, 1.910522504832140594E-31, -5.551115123125818447E-17 ) ) ;
#2605=ADVANCED_FACE ( 'NONE', ( #14780 ), #18763, .T. ) ;
#2620=EDGE_CURVE ( 'NONE', #5493, #22681, #14628, .T. ) ;
#2622=ORIENTED_EDGE ( 'NONE', *, *, #6541, .T. ) ;
#2633=CARTESIAN_POINT ( 'NONE',  ( 7.725871784772784245, -1.814340584914947430, 8.100883686804943196 ) ) ;
#2638=FACE_OUTER_BOUND ( 'NONE', #5699, .T. ) ;
#2644=VERTEX_POINT ( 'NONE', #22776 ) ;
#2648=ORIENTED_EDGE ( 'NONE', *, *, #9543, .T. ) ;
#2660=CARTESIAN_POINT ( 'NONE',  ( -7.876571740167121582, -13.80606002021568735, 7.785394814391164431 ) ) ;
#2668=ORIENTED_EDGE ( 'NONE', *, *, #7782, .T. ) ;
#2669=ORIENTED_EDGE ( 'NONE', *, *, #2077, .T. ) ;
#2683=CARTESIAN_POINT ( 'NONE',  ( -7.500000000000020428, -1.223704156646857388, 9.030675447288954771 ) ) ;
#2706=FACE_OUTER_BOUND ( 'NONE', #18363, .T. ) ;
#2715=CARTESIAN_POINT ( 'NONE',  ( -12.85000000000001386, -12.00000000000006928, 4.163336342344337027E-14 ) ) ;
#2729=DIRECTION ( 'NONE',  ( 1.000000000000000000, 2.168404344971017743E-16, -1.780660105995169760E-30 ) ) ;
#2769=ADVANCED_FACE ( 'NONE', ( #10069 ), #13858, .T. ) ;
#2770=DIRECTION ( 'NONE',  ( 9.121204216617949000E-31, 1.000000000000000000, -6.982962677686261977E-15 ) ) ;
#2775=AXIS2_PLACEMENT_3D ( 'NONE', #1028, #1258, #8197 ) ;
#2777=CIRCLE ( 'NONE', #17813, 2.549999999999997158 ) ;
#2781=CARTESIAN_POINT ( 'NONE',  ( -7.951003271401806849, -13.83829779185615294, 7.659883344695980867 ) ) ;
#2789=EDGE_CURVE ( 'NONE', #10026, #18942, #16089, .T. ) ;
#2791=DIRECTION ( 'NONE',  ( 1.000000000000000000, 6.224605580259554159E-31, -2.887593071917436153E-31 ) ) ;
#2797=EDGE_CURVE ( 'NONE', #6091, #12774, #13476, .T. ) ;
#2812=CARTESIAN_POINT ( 'NONE',  ( -7.500000000000020428, -1.390227771353544473, 9.250000000000008882 ) ) ;
#2815=CARTESIAN_POINT ( 'NONE',  ( -6.999999999999992006, -7.999999999999996447, 11.74999999999999645 ) ) ;
#2820=LINE ( 'NONE', #22935, #20615 ) ;
#2844=DIRECTION ( 'NONE',  ( 0.000000000000000000, 0.000000000000000000, 1.000000000000000000 ) ) ;
#2851=ORIENTED_EDGE ( 'NONE', *, *, #2077, .F. ) ;
#2877=EDGE_LOOP ( 'NONE', ( #3907, #14363, #14882, #229, #11491, #20883 ) ) ;
#2882=DIRECTION ( 'NONE',  ( 0.000000000000000000, 0.000000000000000000, 1.000000000000000000 ) ) ;
#2896=FACE_OUTER_BOUND ( 'NONE', #16298, .T. ) ;
#2897=TOROIDAL_SURFACE ( 'NONE', #16032, 3.500000000000000000, 0.5000000000000000000 ) ;
#2924=CARTESIAN_POINT ( 'NONE',  ( -8.725359747074515226, -0.4999999928004963401, 6.816426071237475348 ) ) ;
#2947=FACE_OUTER_BOUND ( 'NONE', #5917, .T. ) ;
#2952=DIRECTION ( 'NONE',  ( 1.000000000000000000, 1.910522504832140594E-31, -5.551115123125818447E-17 ) ) ;
#2956=AXIS2_PLACEMENT_3D ( 'NONE', #18708, #14833, #22011 ) ;
#2958=EDGE_CURVE ( 'NONE', #10026, #3117, #17998, .T. ) ;
#2959=CARTESIAN_POINT ( 'NONE',  ( -7.000000000000020428, -8.000000000000003553, 12.24999999999999645 ) ) ;
#2962=AXIS2_PLACEMENT_3D ( 'NONE', #1115, #19095, #20524 ) ;
#2963=DIRECTION ( 'NONE',  ( 0.000000000000000000, 0.000000000000000000, 1.000000000000000000 ) ) ;
#2968=ORIENTED_EDGE ( 'NONE', *, *, #10105, .T. ) ;
#2981=CARTESIAN_POINT ( 'NONE',  ( -8.037202331403086930, -2.196591282338350659, 7.528743044528591888 ) ) ;
#2983=DIRECTION ( 'NONE',  ( -9.121204216617949000E-31, -1.000000000000000000, 6.982962677686261977E-15 ) ) ;
#3020=FILL_AREA_STYLE ('',( #11600 ) ) ;
#3022=CARTESIAN_POINT ( 'NONE',  ( 12.84999999999997300, -13.50000000000003020, 5.750000000000047073 ) ) ;
#3050=AXIS2_PLACEMENT_3D ( 'NONE', #14118, #1192, #3307 ) ;
#3061=EDGE_CURVE ( 'NONE', #20416, #16256, #4078, .T. ) ;
#3065=AXIS2_PLACEMENT_3D ( 'NONE', #20550, #11940, #16991 ) ;
#3069=DIRECTION ( 'NONE',  ( -9.121204216617949000E-31, -1.000000000000000000, 6.982962677686261977E-15 ) ) ;
#3081=CIRCLE ( 'NONE', #6087, 5.749999999999992006 ) ;
#3089=ADVANCED_FACE ( 'NONE', ( #2511 ), #15795, .T. ) ;
#3091=ADVANCED_FACE ( 'NONE', ( #10704 ), #12702, .T. ) ;
#3092=FACE_BOUND ( 'NONE', #12650, .T. ) ;
#3093=CARTESIAN_POINT ( 'NONE',  ( 12.84999999999997300, 0.000000000000000000, 1.387778780781445676E-14 ) ) ;
#3097=CARTESIAN_POINT ( 'NONE',  ( -8.697224362268011433, 6.938893903907228378E-15, 6.249999999999992006 ) ) ;
#3098=CARTESIAN_POINT ( 'NONE',  ( -8.422565759993835499, -1.999999999999987121, 6.396710472007108628 ) ) ;
#3099=DIRECTION ( 'NONE',  ( -9.121204216617949000E-31, -1.000000000000000000, 6.982962677686276966E-15 ) ) ;
#3117=VERTEX_POINT ( 'NONE', #5427 ) ;
#3127=CARTESIAN_POINT ( 'NONE',  ( -7.644579933246792969, -13.15747815713137570, 8.321099285265857404 ) ) ;
#3144=AXIS2_PLACEMENT_3D ( 'NONE', #22974, #10258, #17429 ) ;
#3149=VERTEX_POINT ( 'NONE', #19532 ) ;
#3157=AXIS2_PLACEMENT_3D ( 'NONE', #17026, #940, #10642 ) ;
#3160=CARTESIAN_POINT ( 'NONE',  ( 7.000000000000006217, -1.999999999999994893, 10.74999999999998224 ) ) ;
#3163=CARTESIAN_POINT ( 'NONE',  ( -7.499999999999992895, -14.00000000000004441, 6.250000000000047073 ) ) ;
#3180=VERTEX_POINT ( 'NONE', #9178 ) ;
#3224=FACE_BOUND ( 'NONE', #18759, .T. ) ;
#3244=AXIS2_PLACEMENT_3D ( 'NONE', #20977, #10035, #8389 ) ;
#3247=CARTESIAN_POINT ( 'NONE',  ( -7.909386411297020025, -13.36290293203342650, 7.731447622712522616 ) ) ;
#3278=CARTESIAN_POINT ( 'NONE',  ( -7.500000000000024869, -0.9711575687493196885, 9.522727272727292913 ) ) ;
#3294=ORIENTED_EDGE ( 'NONE', *, *, #5491, .T. ) ;
#3307=DIRECTION ( 'NONE',  ( -1.927470528863118556E-16, 1.000000000000000000, -1.252855843761027101E-14 ) ) ;
#3323=ORIENTED_EDGE ( 'NONE', *, *, #15166, .T. ) ;
#3324=ORIENTED_EDGE ( 'NONE', *, *, #353, .T. ) ;
#3329=DIRECTION ( 'NONE',  ( 0.000000000000000000, -7.888609052210128564E-31, 1.000000000000000000 ) ) ;
#3344=DIRECTION ( 'NONE',  ( 0.000000000000000000, 6.938893903907245733E-15, 1.000000000000000000 ) ) ;
#3346=CARTESIAN_POINT ( 'NONE',  ( 10.50000000000000888, -14.00000000000003020, 5.750000000000047073 ) ) ;
#3347=DIRECTION ( 'NONE',  ( -9.121204216617949000E-31, -1.000000000000000000, 6.982962677686261977E-15 ) ) ;
#3349=DIRECTION ( 'NONE',  ( 0.000000000000000000, 0.000000000000000000, -1.000000000000000000 ) ) ;
#3350=( GEOMETRIC_REPRESENTATION_CONTEXT ( 3 ) GLOBAL_UNCERTAINTY_ASSIGNED_CONTEXT ( ( #13328 ) ) GLOBAL_UNIT_ASSIGNED_CONTEXT ( ( #22674, #15238, #21022 ) ) REPRESENTATION_CONTEXT ( 'NONE', 'WORKASPACE' ) );
#3351=VERTEX_POINT ( 'NONE', #14925 ) ;
#3358=EDGE_LOOP ( 'NONE', ( #20124, #21694, #4218, #3491 ) ) ;
#3360=AXIS2_PLACEMENT_3D ( 'NONE', #9607, #211, #5969 ) ;
#3372=CARTESIAN_POINT ( 'NONE',  ( -7.644579933246753001, -0.8425218428686375161, 8.321099285265791679 ) ) ;
#3391=CARTESIAN_POINT ( 'NONE',  ( 7.786490775660112718, -0.7065074219475176998, 7.963863235126067863 ) ) ;
#3393=CYLINDRICAL_SURFACE ( 'NONE', #12644, 0.4999999999999987232 ) ;
#3398=CARTESIAN_POINT ( 'NONE',  ( -8.178874953434677408, -0.007851515978185664296, 6.644730819938938104 ) ) ;
#3406=VERTEX_POINT ( 'NONE', #22931 ) ;
#3422=CARTESIAN_POINT ( 'NONE',  ( -6.999999999999992006, -13.02884243125069652, 9.522727272727321335 ) ) ;
#3431=EDGE_LOOP ( 'NONE', ( #6975, #7910, #4809, #2968 ) ) ;
#3440=CARTESIAN_POINT ( 'NONE',  ( -8.697224362268011433, -12.00000000000004263, 6.250000000000019540 ) ) ;
#3443=CARTESIAN_POINT ( 'NONE',  ( 12.84999999999997300, -12.00000000000006928, 4.163336342344337027E-14 ) ) ;
#3444=DIRECTION ( 'NONE',  ( 1.454462294001240516E-30, 1.000000000000000000, 0.000000000000000000 ) ) ;
#3447=CARTESIAN_POINT ( 'NONE',  ( -10.49999999999999467, -12.00000000000000711, 9.250000000000021316 ) ) ;
#3450=CARTESIAN_POINT ( 'NONE',  ( 7.862302507584130851, -2.046564842090945913, 6.866983975782614102 ) ) ;
#3451=CIRCLE ( 'NONE', #16569, 3.499999999999995115 ) ;
#3454=ORIENTED_EDGE ( 'NONE', *, *, #4753, .F. ) ;
#3491=ORIENTED_EDGE ( 'NONE', *, *, #8983, .F. ) ;
#3492=EDGE_CURVE ( 'NONE', #15314, #16729, #20217, .T. ) ;
#3497=DIRECTION ( 'NONE',  ( -1.734723475976813750E-16, -1.000000000000000000, 3.469446951953607484E-15 ) ) ;
#3502=FACE_OUTER_BOUND ( 'NONE', #8907, .T. ) ;
#3516=EDGE_CURVE ( 'NONE', #6724, #14530, #13864, .T. ) ;
#3521=TOROIDAL_SURFACE ( 'NONE', #15164, 5.750000000000000000, 0.5000000000000000000 ) ;
#3523=EDGE_CURVE ( 'NONE', #20968, #9827, #7435, .T. ) ;
#3531=DIRECTION ( 'NONE',  ( -2.168404344970994323E-16, 1.000000000000000000, -1.577721810442023611E-30 ) ) ;
#3541=CARTESIAN_POINT ( 'NONE',  ( 8.723547172042470876, -2.015988055643229693, 6.817515300135711165 ) ) ;
#3560=CARTESIAN_POINT ( 'NONE',  ( 7.120027569165137571, -11.54977705885981898, 8.099087005775212234 ) ) ;
#3561=CARTESIAN_POINT ( 'NONE',  ( -7.862302507584129074, -11.95343515790908206, 6.866983975782633642 ) ) ;
#3563=( BOUNDED_SURFACE ( )  B_SPLINE_SURFACE ( 3, 2, ( 
 ( #3684, #12736, #508 ),
 ( #21579, #7561, #16589 ),
 ( #17924, #18045, #3906 ),
 ( #4019, #18155, #7679 ),
 ( #16368, #16484, #11201 ),
 ( #12974, #18384, #5459 ),
 ( #18265, #2260, #392 ),
 ( #5572, #9441, #14849 ),
 ( #8986, #10854, #22023 ),
 ( #14726, #9329, #16250 ),
 ( #5911, #167, #12615 ),
 ( #21691, #21918, #13085 ),
 ( #1800, #2026, #270 ),
 ( #9212, #2138, #16138 ) ),
 .UNSPECIFIED., .F., .F., .T. ) 
 B_SPLINE_SURFACE_WITH_KNOTS ( ( 4, 2, 2, 2, 2, 2, 4 ),
 ( 3, 3 ),
 ( -2.168404344971008868E-19, 0.0009385527998839222766, 0.001407829199825883469, 0.001877105599767844770, 0.002346381999709806071, 0.002815658399651766938, 0.003754211199535689540 ),
 ( 0.000000000000000000, 1.000000000000000000 ),
 .UNSPECIFIED. ) 
 GEOMETRIC_REPRESENTATION_ITEM ( )  RATIONAL_B_SPLINE_SURFACE ( (
 ( 1.000000000000000000, 0.7071067811865494601, 1.000000000000000000),
 ( 1.000000000000000000, 0.7217349950159032135, 1.000000000000000000),
 ( 1.000000000000000000, 0.7325631490737081197, 1.000000000000000000),
 ( 1.000000000000000000, 0.7426392126583249986, 1.000000000000000000),
 ( 1.000000000000000000, 0.7449451721693722828, 1.000000000000000000),
 ( 1.000000000000000000, 0.7474053618998901527, 1.000000000000000000),
 ( 1.000000000000000000, 0.7475947887410621107, 1.000000000000000000),
 ( 1.000000000000000000, 0.7461109904165270645, 1.000000000000000000),
 ( 1.000000000000000000, 0.7444113185333118832, 1.000000000000000000),
 ( 1.000000000000000000, 0.7395217850810087423, 1.000000000000000000),
 ( 1.000000000000000000, 0.7363545993504165832, 1.000000000000000000),
 ( 1.000000000000000000, 0.7253814056385120557, 1.000000000000000000),
 ( 1.000000000000000000, 0.7159765610437058836, 1.000000000000000000),
 ( 1.000000000000000000, 0.7071067811865503483, 1.000000000000000000) ) ) 
 REPRESENTATION_ITEM ( '' )  SURFACE ( )  );
#3564=CARTESIAN_POINT ( 'NONE',  ( 7.980290731945721916, -13.39170085596636461, 7.616182555102830598 ) ) ;
#3570=DIRECTION ( 'NONE',  ( 0.000000000000000000, 0.000000000000000000, 1.000000000000000000 ) ) ;
#3572=DIRECTION ( 'NONE',  ( -1.000000000000000000, -1.910522504832140594E-31, 5.551115123125818447E-17 ) ) ;
#3578=ORIENTED_EDGE ( 'NONE', *, *, #18112, .F. ) ;
#3581=ORIENTED_EDGE ( 'NONE', *, *, #21643, .T. ) ;
#3585=ORIENTED_EDGE ( 'NONE', *, *, #18079, .F. ) ;
#3602=CARTESIAN_POINT ( 'NONE',  ( 12.84999999999997300, -1.500000000000001332, 6.250000000000005329 ) ) ;
#3607=ORIENTED_EDGE ( 'NONE', *, *, #1466, .F. ) ;
#3609=AXIS2_PLACEMENT_3D ( 'NONE', #2203, #3843, #13256 ) ;
#3610=EDGE_CURVE ( 'NONE', #21919, #9975, #18693, .T. ) ;
#3666=CARTESIAN_POINT ( 'NONE',  ( 7.734741761309930297, -11.93000978614839269, 7.004299047562712488 ) ) ;
#3684=CARTESIAN_POINT ( 'NONE',  ( 7.500000000000007105, -1.390227771353540698, 9.250000000000019540 ) ) ;
#3690=ORIENTED_EDGE ( 'NONE', *, *, #8234, .T. ) ;
#3698=ADVANCED_FACE ( 'NONE', ( #20551 ), #12911, .T. ) ;
#3713=ORIENTED_EDGE ( 'NONE', *, *, #617, .T. ) ;
#3716=ORIENTED_EDGE ( 'NONE', *, *, #20136, .T. ) ;
#3724=LINE ( 'NONE', #7162, #17320 ) ;
#3729=DIRECTION ( 'NONE',  ( -9.121204216617949000E-31, -1.000000000000000000, 6.982962677686261977E-15 ) ) ;
#3731=CARTESIAN_POINT ( 'NONE',  ( -12.85000000000001386, -13.50000000000007105, 5.551115123125782702E-14 ) ) ;
#3737=DIRECTION ( 'NONE',  ( 0.000000000000000000, 6.938893903907237055E-15, 1.000000000000000000 ) ) ;
#3739=ORIENTED_EDGE ( 'NONE', *, *, #18079, .T. ) ;
#3741=CARTESIAN_POINT ( 'NONE',  ( 12.84999999999997300, -1.500000000000001332, -6.249999999999977796 ) ) ;
#3747=ORIENTED_EDGE ( 'NONE', *, *, #22340, .T. ) ;
#3752=CARTESIAN_POINT ( 'NONE',  ( 7.742458795615099199, -13.26006887186488292, 8.061568688626010726 ) ) ;
#3759=AXIS2_PLACEMENT_3D ( 'NONE', #14371, #14710, #16235 ) ;
#3760=ORIENTED_EDGE ( 'NONE', *, *, #18965, .F. ) ;
#3772=CARTESIAN_POINT ( 'NONE',  ( 7.467942433933819402, -11.84606835491525878, 7.356484134531164898 ) ) ;
#3774=CARTESIAN_POINT ( 'NONE',  ( -7.026577802269679651, -11.35109376985337981, 8.453373545151620760 ) ) ;
#3784=ADVANCED_FACE ( 'NONE', ( #22901, #9841, #4770 ), #13941, .T. ) ;
#3788=FACE_OUTER_BOUND ( 'NONE', #18046, .T. ) ;
#3794=ORIENTED_EDGE ( 'NONE', *, *, #4921, .T. ) ;
#3803=DIRECTION ( 'NONE',  ( -9.121204216617949000E-31, -1.000000000000000000, 6.982962677686261977E-15 ) ) ;
#3831=CIRCLE ( 'NONE', #5365, 0.4999999999999987232 ) ;
#3833=CARTESIAN_POINT ( 'NONE',  ( 12.84999999999997300, -1.999999999999998224, 0.000000000000000000 ) ) ;
#3834=DIRECTION ( 'NONE',  ( 1.000000000000000000, -2.312964634635739999E-16, 1.302601544865244959E-30 ) ) ;
#3840=CARTESIAN_POINT ( 'NONE',  ( 7.764145988665074327, -1.774864566462285520, 8.011880279048840592 ) ) ;
#3843=DIRECTION ( 'NONE',  ( -1.000000000000000000, -1.910522504832140594E-31, 5.551115123125818447E-17 ) ) ;
#3859=CARTESIAN_POINT ( 'NONE',  ( 12.84999999999997300, -14.00000000000011369, -5.749999999999921840 ) ) ;
#3865=CARTESIAN_POINT ( 'NONE',  ( 7.000000000000020428, -13.02884243125069652, 9.522727272727321335 ) ) ;
#3867=CARTESIAN_POINT ( 'NONE',  ( 7.479729963978305918, -13.19653517305387780, 9.265052153035679083 ) ) ;
#3888=VECTOR ( 'NONE', #3729, 1000.000000000000000 ) ;
#3899=DIRECTION ( 'NONE',  ( 0.000000000000000000, 0.000000000000000000, 1.000000000000000000 ) ) ;
#3906=CARTESIAN_POINT ( 'NONE',  ( 7.029812747553613406, -0.6228290751908035494, 8.933015330925462294 ) ) ;
#3907=ORIENTED_EDGE ( 'NONE', *, *, #10827, .T. ) ;
#3908=AXIS2_PLACEMENT_3D ( 'NONE', #7894, #11418, #16579 ) ;
#3916=ORIENTED_EDGE ( 'NONE', *, *, #21643, .F. ) ;
#3944=ORIENTED_EDGE ( 'NONE', *, *, #22340, .F. ) ;
#3955=CARTESIAN_POINT ( 'NONE',  ( 12.84999999999997300, -1.999999999999998224, 0.000000000000000000 ) ) ;
#3956=ADVANCED_FACE ( 'NONE', ( #12522 ), #20261, .T. ) ;
#3958=CARTESIAN_POINT ( 'NONE',  ( -7.761744141695535504, -2.064358047808336316, 6.973942750959534642 ) ) ;
#3963=DIRECTION ( 'NONE',  ( 1.577021341797097314E-16, 1.000000000000000000, -1.734723475976807094E-15 ) ) ;
#3969=CIRCLE ( 'NONE', #22758, 0.4999999999999995559 ) ;
#3978=CYLINDRICAL_SURFACE ( 'NONE', #19896, 0.4999999999999995559 ) ;
#3979=CARTESIAN_POINT ( 'NONE',  ( -12.85000000000001386, -13.50000000000007105, 5.551115123125782702E-14 ) ) ;
#3982=CARTESIAN_POINT ( 'NONE',  ( 7.271441198316241916, -13.72907106061213511, 8.039702399269780031 ) ) ;
#3988=FILL_AREA_STYLE ('',( #711 ) ) ;
#3989=EDGE_CURVE ( 'NONE', #138, #10463, #16161, .T. ) ;
#3991=CIRCLE ( 'NONE', #11869, 0.4999999999999992228 ) ;
#4001=CARTESIAN_POINT ( 'NONE',  ( 7.000000000000006217, -0.9711575687493152476, 9.522727272727294690 ) ) ;
#4002=CARTESIAN_POINT ( 'NONE',  ( 7.710998176012808791, -11.54387914083316424, 8.114728912742409150 ) ) ;
#4010=CARTESIAN_POINT ( 'NONE',  ( 8.697224362267983011, -1.999999999999984457, 6.249999999999992006 ) ) ;
#4019=CARTESIAN_POINT ( 'NONE',  ( 7.613388670473284492, -0.8883455870200749338, 8.423574099071707622 ) ) ;
#4026=EDGE_LOOP ( 'NONE', ( #10568, #22388, #18994, #18617 ) ) ;
#4034=ORIENTED_EDGE ( 'NONE', *, *, #6957, .F. ) ;
#4042=AXIS2_PLACEMENT_3D ( 'NONE', #13320, #5809, #6028 ) ;
#4049=CARTESIAN_POINT ( 'NONE',  ( 10.50000000000000888, -0.5000000000000004441, 9.250000000000008882 ) ) ;
#4058=VECTOR ( 'NONE', #20823, 1000.000000000000000 ) ;
#4060=ORIENTED_EDGE ( 'NONE', *, *, #9572, .F. ) ;
#4074=CARTESIAN_POINT ( 'NONE',  ( -7.734741761309930297, -11.93000978614838559, 7.004299047562723146 ) ) ;
#4075=CARTESIAN_POINT ( 'NONE',  ( -7.479729963973698936, -13.19653517305877166, 9.265052153039251337 ) ) ;
#4078=CIRCLE ( 'NONE', #2962, 0.4999999999999995559 ) ;
#4079=CARTESIAN_POINT ( 'NONE',  ( 8.832214555408109291, -1.499999999999984457, 6.752214322824766413 ) ) ;
#4080=CYLINDRICAL_SURFACE ( 'NONE', #3609, 0.4999999999999995559 ) ;
#4087=DIRECTION ( 'NONE',  ( 2.168404344970994323E-16, -1.000000000000000000, 1.577721810442023611E-30 ) ) ;
#4095=CARTESIAN_POINT ( 'NONE',  ( -12.84999999999999964, -0.5000000000000004441, -5.749999999999963585 ) ) ;
#4108=EDGE_LOOP ( 'NONE', ( #3739, #20862, #14959, #13007 ) ) ;
#4129=CARTESIAN_POINT ( 'NONE',  ( 6.999999999999978684, -2.818969682667037624, 8.693499985977959810 ) ) ;
#4151=CARTESIAN_POINT ( 'NONE',  ( -7.523705677352342747, -2.838350495272803364, 8.715168381933473540 ) ) ;
#4155=CYLINDRICAL_SURFACE ( 'NONE', #7231, 5.999999999999991118 ) ;
#4173=ORIENTED_EDGE ( 'NONE', *, *, #1392, .F. ) ;
#4179=CARTESIAN_POINT ( 'NONE',  ( -7.638377885296727676, -12.06377841978599363, 8.340398698103474118 ) ) ;
#4181=CARTESIAN_POINT ( 'NONE',  ( -7.742458795615090317, -13.26006887186487937, 8.061568688626005397 ) ) ;
#4199=EDGE_CURVE ( 'NONE', #2238, #19516, #11678, .T. ) ;
#4201=DIRECTION ( 'NONE',  ( -4.019602852144215652E-47, -6.982962677686261977E-15, -1.000000000000000000 ) ) ;
#4205=CIRCLE ( 'NONE', #20761, 2.549999999999997158 ) ;
#4206=CARTESIAN_POINT ( 'NONE',  ( 7.028413389564970970, -13.36994781876315486, 8.946655872546040555 ) ) ;
#4207=DIRECTION ( 'NONE',  ( 0.000000000000000000, 0.000000000000000000, -1.000000000000000000 ) ) ;
#4218=ORIENTED_EDGE ( 'NONE', *, *, #16575, .F. ) ;
#4219=CIRCLE ( 'NONE', #15511, 0.4999999999999995559 ) ;
#4222=ORIENTED_EDGE ( 'NONE', *, *, #14818, .F. ) ;
#4242=LINE ( 'NONE', #7902, #14224 ) ;
#4256=CARTESIAN_POINT ( 'NONE',  ( -12.84999999999999964, -2.000000000000001776, 0.000000000000000000 ) ) ;
#4271=DIRECTION ( 'NONE',  ( -1.000000000000000000, -2.168404344971017743E-16, 1.780660105995169760E-30 ) ) ;
#4275=DIRECTION ( 'NONE',  ( -9.121204216617949000E-31, -1.000000000000000000, 6.982962677686261977E-15 ) ) ;
#4286=ORIENTED_EDGE ( 'NONE', *, *, #7371, .F. ) ;
#4294=DIRECTION ( 'NONE',  ( 0.000000000000000000, 0.000000000000000000, 1.000000000000000000 ) ) ;
#4296=CARTESIAN_POINT ( 'NONE',  ( -7.972478112619585389, -12.36350260656811528, 7.628219499134346826 ) ) ;
#4298=CARTESIAN_POINT ( 'NONE',  ( -8.178874953434455364, -13.99214848402183087, 6.644730819939131727 ) ) ;
#4334=ORIENTED_EDGE ( 'NONE', *, *, #11549, .T. ) ;
#4340=MECHANICAL_DESIGN_GEOMETRIC_PRESENTATION_REPRESENTATION('',(#22773),#12617);
#4343=VERTEX_POINT ( 'NONE', #3346 ) ;
#4372=EDGE_LOOP ( 'NONE', ( #398, #20998, #14486, #5957 ) ) ;
#4375=DIRECTION ( 'NONE',  ( 0.000000000000000000, 6.802837160693368935E-15, 1.000000000000000000 ) ) ;
#4390=PRODUCT_DEFINITION_SHAPE ( 'NONE', 'NONE',  #15220 ) ;
#4396=AXIS2_PLACEMENT_3D ( 'NONE', #17120, #20805, #17241 ) ;
#4401=EDGE_CURVE ( 'NONE', #18942, #15314, #21461, .T. ) ;
#4409=FACE_OUTER_BOUND ( 'NONE', #15968, .T. ) ;
#4414=CARTESIAN_POINT ( 'NONE',  ( -8.498922697886669653, -12.49080420435820926, 6.997949321565080538 ) ) ;
#4415=VECTOR ( 'NONE', #19101, 1000.000000000000000 ) ;
#4423=AXIS2_PLACEMENT_3D ( 'NONE', #19535, #21437, #1662 ) ;
#4435=DIRECTION ( 'NONE',  ( 1.454462294001240516E-30, 1.000000000000000000, 0.000000000000000000 ) ) ;
#4454=EDGE_CURVE ( 'NONE', #9571, #5465, #16022, .T. ) ;
#4455=CARTESIAN_POINT ( 'NONE',  ( -12.84999999999999964, -12.00000000000011191, -5.749999999999963585 ) ) ;
#4473=EDGE_CURVE ( 'NONE', #22681, #9370, #22052, .T. ) ;
#4479=DIRECTION ( 'NONE',  ( 0.000000000000000000, -0.7453559924999264563, 0.6666666666666704044 ) ) ;
#4481=EDGE_CURVE ( 'NONE', #396, #4924, #17145, .T. ) ;
#4482=DIRECTION ( 'NONE',  ( 1.454462294001240516E-30, 1.000000000000000000, 0.000000000000000000 ) ) ;
#4501=EDGE_CURVE ( 'NONE', #17483, #16256, #7033, .T. ) ;
#4504=DIRECTION ( 'NONE',  ( 1.000000000000000000, 6.224605580259554159E-31, -2.887593071917436153E-31 ) ) ;
#4510=CARTESIAN_POINT ( 'NONE',  ( 8.037202331403262789, -2.196591282338120621, 7.528743044528568795 ) ) ;
#4511=LINE ( 'NONE', #22399, #538 ) ;
#4522=ORIENTED_EDGE ( 'NONE', *, *, #12794, .F. ) ;
#4536=CARTESIAN_POINT ( 'NONE',  ( -10.49999999999998224, -12.00000000000002842, 5.750000000000018652 ) ) ;
#4538=CARTESIAN_POINT ( 'NONE',  ( -8.429621201837608879, -14.00000000000004619, 6.425428529985135917 ) ) ;
#4551=ORIENTED_EDGE ( 'NONE', *, *, #11549, .F. ) ;
#4588=DIRECTION ( 'NONE',  ( -9.121204216617949000E-31, -1.000000000000000000, 6.982962677686261977E-15 ) ) ;
#4600=EDGE_LOOP ( 'NONE', ( #12470, #7198, #22125, #11896 ) ) ;
#4617=AXIS2_PLACEMENT_3D ( 'NONE', #1105, #2729, #13904 ) ;
#4626=CARTESIAN_POINT ( 'NONE',  ( -10.49999999999999467, -12.00000000000000711, 9.250000000000021316 ) ) ;
#4661=CARTESIAN_POINT ( 'NONE',  ( -8.496394830447192348, -13.96748264593578526, 6.998792816379799220 ) ) ;
#4668=DIRECTION ( 'NONE',  ( 1.000000000000000000, 2.168404344971017743E-16, -1.780660105995169760E-30 ) ) ;
#4683=FACE_OUTER_BOUND ( 'NONE', #18648, .T. ) ;
#4688=CARTESIAN_POINT ( 'NONE',  ( -8.721922330811995749, -0.01237189218572515466, 6.818491697977000499 ) ) ;
#4690=CARTESIAN_POINT ( 'NONE',  ( 8.697224362267995446, -14.00000000000004974, 6.250000000000070166 ) ) ;
#4695=CARTESIAN_POINT ( 'NONE',  ( -7.500000000000020428, -1.390227771353544473, 9.250000000000008882 ) ) ;
#4710=ORIENTED_EDGE ( 'NONE', *, *, #11545, .F. ) ;
#4727=ORIENTED_EDGE ( 'NONE', *, *, #8358, .T. ) ;
#4740=CARTESIAN_POINT ( 'NONE',  ( 8.129778652391200566, -1.578738987863736565, 7.405931224841482141 ) ) ;
#4753=EDGE_CURVE ( 'NONE', #5440, #19516, #3969, .T. ) ;
#4770=FACE_OUTER_BOUND ( 'NONE', #10832, .T. ) ;
#4775=ADVANCED_FACE ( 'NONE', ( #8802 ), #15957, .T. ) ;
#4785=ORIENTED_EDGE ( 'NONE', *, *, #7109, .F. ) ;
#4787=DIRECTION ( 'NONE',  ( 2.478176394252584494E-15, -7.888609052210165348E-31, 1.000000000000000000 ) ) ;
#4792=VECTOR ( 'NONE', #12564, 1000.000000000000000 ) ;
#4797=CARTESIAN_POINT ( 'NONE',  ( -7.651206356577011647, -0.8338323182647964238, 8.300907142094176905 ) ) ;
#4801=AXIS2_PLACEMENT_3D ( 'NONE', #20267, #11199, #18836 ) ;
#4805=CARTESIAN_POINT ( 'NONE',  ( -10.49999999999998224, -12.00000000000002842, 5.750000000000018652 ) ) ;
#4809=ORIENTED_EDGE ( 'NONE', *, *, #19052, .F. ) ;
#4817=CARTESIAN_POINT ( 'NONE',  ( 7.500000000000007105, -8.000000000000010658, 10.75000000000000888 ) ) ;
#4847=CIRCLE ( 'NONE', #12742, 2.999999999999995559 ) ;
#4863=VERTEX_POINT ( 'NONE', #14664 ) ;
#4869=FACE_OUTER_BOUND ( 'NONE', #8868, .T. ) ;
#4870=CARTESIAN_POINT ( 'NONE',  ( -7.499999999999992895, -8.000000000000044409, 6.250000000000005329 ) ) ;
#4900=FACE_OUTER_BOUND ( 'NONE', #9767, .T. ) ;
#4905=FACE_OUTER_BOUND ( 'NONE', #8751, .T. ) ;
#4921=EDGE_CURVE ( 'NONE', #21322, #11731, #3991, .T. ) ;
#4924=VERTEX_POINT ( 'NONE', #9961 ) ;
#4934=ADVANCED_FACE ( 'NONE', ( #9727 ), #20635, .T. ) ;
#4938=DIRECTION ( 'NONE',  ( -4.019602852144232182E-47, -6.982962677686261977E-15, -1.000000000000000000 ) ) ;
#4939=DIRECTION ( 'NONE',  ( -1.577021341797097314E-16, 1.000000000000000000, -3.627149086133324068E-15 ) ) ;
#4943=CARTESIAN_POINT ( 'NONE',  ( 0.000000000000000000, 0.000000000000000000, 0.000000000000000000 ) ) ;
#4953=ORIENTED_EDGE ( 'NONE', *, *, #17828, .T. ) ;
#4970=EDGE_CURVE ( 'NONE', #19164, #18123, #15252, .T. ) ;
#4971=CIRCLE ( 'NONE', #20780, 2.549999999999997158 ) ;
#4992=EDGE_LOOP ( 'NONE', ( #2465, #21053, #12686, #11509 ) ) ;
#5007=AXIS2_PLACEMENT_3D ( 'NONE', #20281, #6162, #2150 ) ;
#5020=( BOUNDED_SURFACE ( )  B_SPLINE_SURFACE ( 3, 2, ( 
 ( #14261, #14368, #255 ),
 ( #9309, #21675, #20128 ),
 ( #5555, #20013, #19670 ),
 ( #12954, #10721, #3560 ),
 ( #17908, #4002, #12721 ),
 ( #12602, #19906, #39 ),
 ( #7432, #19787, #21450 ),
 ( #21790, #2246, #3772 ),
 ( #1888, #18250, #2121 ),
 ( #14706, #14603, #3666 ),
 ( #10838, #21896, #9073 ),
 ( #10941, #16572, #2007 ),
 ( #16232, #150, #18369 ),
 ( #9196, #22366, #9541 ) ),
 .UNSPECIFIED., .F., .F., .T. ) 
 B_SPLINE_SURFACE_WITH_KNOTS ( ( 4, 2, 2, 2, 2, 2, 4 ),
 ( 3, 3 ),
 ( 0.000000000000000000, 0.0009656398008937971521, 0.001448459701340695620, 0.001931279601787594304, 0.002414099502234492989, 0.002896919402681391240, 0.003862559203575188609 ),
 ( 0.000000000000000000, 1.000000000000000000 ),
 .UNSPECIFIED. ) 
 GEOMETRIC_REPRESENTATION_ITEM ( )  RATIONAL_B_SPLINE_SURFACE ( (
 ( 1.000000000000000000, 0.7071067811865429098, 1.000000000000000000),
 ( 1.000000000000000000, 0.6907538105667043737, 1.000000000000000000),
 ( 1.000000000000000000, 0.6765417438350033175, 1.000000000000000000),
 ( 1.000000000000000000, 0.6623232117678236053, 1.000000000000000000),
 ( 1.000000000000000000, 0.6588386061805659999, 1.000000000000000000),
 ( 1.000000000000000000, 0.6547992448372328411, 1.000000000000000000),
 ( 1.000000000000000000, 0.6542040191408873273, 1.000000000000000000),
 ( 1.000000000000000000, 0.6557724471762160778, 1.000000000000000000),
 ( 1.000000000000000000, 0.6579729115737033007, 1.000000000000000000),
 ( 1.000000000000000000, 0.6644691908065228914, 1.000000000000000000),
 ( 1.000000000000000000, 0.6687559023949211090, 1.000000000000000000),
 ( 1.000000000000000000, 0.6835702420294266224, 1.000000000000000000),
 ( 1.000000000000000000, 0.6960226107070131008, 1.000000000000000000),
 ( 1.000000000000000000, 0.7071067811865431318, 1.000000000000000000) ) ) 
 REPRESENTATION_ITEM ( '' )  SURFACE ( )  );
#5022=CARTESIAN_POINT ( 'NONE',  ( 7.523653856849480626, -1.079621694564734780, 8.801128846369474346 ) ) ;
#5024=TOROIDAL_SURFACE ( 'NONE', #11399, 4.500000000000000888, 0.5000000000000000000 ) ;
#5034=DIRECTION ( 'NONE',  ( 1.577021341797097314E-16, 1.000000000000000000, 0.000000000000000000 ) ) ;
#5041=DIRECTION ( 'NONE',  ( 1.000000000000000000, 0.000000000000000000, 0.000000000000000000 ) ) ;
#5045=ORIENTED_EDGE ( 'NONE', *, *, #21414, .T. ) ;
#5066=DIRECTION ( 'NONE',  ( 9.121204216617949000E-31, 1.000000000000000000, -6.982962677686261977E-15 ) ) ;
#5097=CARTESIAN_POINT ( 'NONE',  ( 7.500000000000007105, -1.999999999999991340, 11.74999999999998224 ) ) ;
#5103=EDGE_LOOP ( 'NONE', ( #1044, #3324 ) ) ;
#5107=ORIENTED_EDGE ( 'NONE', *, *, #17085, .F. ) ;
#5122=CARTESIAN_POINT ( 'NONE',  ( 12.84999999999997300, -1.999999999999998224, 0.000000000000000000 ) ) ;
#5127=EDGE_LOOP ( 'NONE', ( #13263, #19061 ) ) ;
#5133=ORIENTED_EDGE ( 'NONE', *, *, #7820, .F. ) ;
#5135=AXIS2_PLACEMENT_3D ( 'NONE', #12789, #7504, #3963 ) ;
#5149=CARTESIAN_POINT ( 'NONE',  ( -8.233775472210618673, -0.5437072270125806739, 7.279685395985805663 ) ) ;
#5188=AXIS2_PLACEMENT_3D ( 'NONE', #17559, #13806, #20990 ) ;
#5198=ORIENTED_EDGE ( 'NONE', *, *, #9964, .T. ) ;
#5207=DIRECTION ( 'NONE',  ( 0.000000000000000000, 6.802837160693368935E-15, 1.000000000000000000 ) ) ;
#5210=CARTESIAN_POINT ( 'NONE',  ( -7.735962016526085172, -0.06991241830943269175, 7.174192622766982552 ) ) ;
#5211=( BOUNDED_SURFACE ( )  B_SPLINE_SURFACE ( 3, 2, ( 
 ( #8455, #3278, #19151 ),
 ( #10324, #13631, #10445 ),
 ( #15381, #8331, #19379 ),
 ( #1509, #6578, #10102 ),
 ( #8223, #17495, #4797 ),
 ( #14089, #20825, #1168 ),
 ( #17372, #15496, #21043 ),
 ( #1285, #19260, #8568 ),
 ( #11968, #6926, #21276 ),
 ( #22569, #22925, #8679 ),
 ( #15614, #12313, #5149 ),
 ( #3398, #22806, #13749 ),
 ( #10203, #4688, #2924 ),
 ( #19502, #20930, #6687 ) ),
 .UNSPECIFIED., .F., .F., .T. ) 
 B_SPLINE_SURFACE_WITH_KNOTS ( ( 4, 2, 2, 2, 2, 2, 4 ),
 ( 3, 3 ),
 ( 1.951563910473907981E-18, 0.0009385527998839240113, 0.001407829199825884987, 0.001877105599767846071, 0.002346381999709806938, 0.002815658399651768239, 0.003754211199535690408 ),
 ( 0.000000000000000000, 1.000000000000000000 ),
 .UNSPECIFIED. ) 
 GEOMETRIC_REPRESENTATION_ITEM ( )  RATIONAL_B_SPLINE_SURFACE ( (
 ( 1.000000000000000000, 0.7071067811865440200, 1.000000000000000000),
 ( 1.000000000000000000, 0.7217349950159128724, 1.000000000000000000),
 ( 1.000000000000000000, 0.7325631490736875806, 1.000000000000000000),
 ( 1.000000000000000000, 0.7426392126583306608, 1.000000000000000000),
 ( 1.000000000000000000, 0.7449451721693339801, 1.000000000000000000),
 ( 1.000000000000000000, 0.7474053618999215720, 1.000000000000000000),
 ( 1.000000000000000000, 0.7475947887410936410, 1.000000000000000000),
 ( 1.000000000000000000, 0.7461109904164890949, 1.000000000000000000),
 ( 1.000000000000000000, 0.7444113185332733584, 1.000000000000000000),
 ( 1.000000000000000000, 0.7395217850810403837, 1.000000000000000000),
 ( 1.000000000000000000, 0.7363545993504035936, 1.000000000000000000),
 ( 1.000000000000000000, 0.7253814056385251563, 1.000000000000000000),
 ( 1.000000000000000000, 0.7159765610436893413, 1.000000000000000000),
 ( 1.000000000000000000, 0.7071067811865459074, 1.000000000000000000) ) ) 
 REPRESENTATION_ITEM ( '' )  SURFACE ( )  );
#5221=CYLINDRICAL_SURFACE ( 'NONE', #8731, 2.999999999999995559 ) ;
#5234=EDGE_LOOP ( 'NONE', ( #15456, #12007, #12891, #16771 ) ) ;
#5237=ORIENTED_EDGE ( 'NONE', *, *, #7076, .F. ) ;
#5247=LINE ( 'NONE', #14179, #10999 ) ;
#5252=AXIS2_PLACEMENT_3D ( 'NONE', #3443, #164, #3737 ) ;
#5262=ORIENTED_EDGE ( 'NONE', *, *, #6541, .F. ) ;
#5270=CARTESIAN_POINT ( 'NONE',  ( 12.84999999999997300, -14.00000000000007105, 5.551115123125782702E-14 ) ) ;
#5277=CARTESIAN_POINT ( 'NONE',  ( -12.85000000000001386, -1.499999999999997780, -5.749999999999976907 ) ) ;
#5279=ADVANCED_FACE ( 'NONE', ( #14754 ), #4155, .T. ) ;
#5306=DIRECTION ( 'NONE',  ( 1.000000000000000000, 0.000000000000000000, 0.000000000000000000 ) ) ;
#5315=CIRCLE ( 'NONE', #7202, 3.499999999999996003 ) ;
#5320=CARTESIAN_POINT ( 'NONE',  ( -12.85000000000001386, -12.00000000000006928, 4.163336342344337027E-14 ) ) ;
#5322=CARTESIAN_POINT ( 'NONE',  ( -7.835312244869949261, -0.05103360697234399224, 7.041165740960511954 ) ) ;
#5323=CARTESIAN_POINT ( 'NONE',  ( 7.523653856849481514, -12.92037830543529253, 8.801128846369500991 ) ) ;
#5331=CARTESIAN_POINT ( 'NONE',  ( 7.162073728446656240, -2.365283217609523092, 7.945145523438303492 ) ) ;
#5343=EDGE_LOOP ( 'NONE', ( #10627, #1078, #6817, #22910 ) ) ;
#5344=ORIENTED_EDGE ( 'NONE', *, *, #16549, .T. ) ;
#5347=ORIENTED_EDGE ( 'NONE', *, *, #2196, .T. ) ;
#5360=DIRECTION ( 'NONE',  ( 1.454462294001240516E-30, 1.000000000000000000, 0.000000000000000000 ) ) ;
#5365=AXIS2_PLACEMENT_3D ( 'NONE', #18989, #6861, #3344 ) ;
#5368=CARTESIAN_POINT ( 'NONE',  ( -7.764145988665025477, -1.774864566462279081, 8.011880279048810394 ) ) ;
#5374=CIRCLE ( 'NONE', #18881, 6.249999999999992006 ) ;
#5389=EDGE_CURVE ( 'NONE', #20148, #20452, #3831, .T. ) ;
#5395=CARTESIAN_POINT ( 'NONE',  ( 7.500000000000007105, -11.35410196624971491, 9.250000000000021316 ) ) ;
#5410=EDGE_CURVE ( 'NONE', #1155, #13674, #17084, .T. ) ;
#5412=AXIS2_PLACEMENT_3D ( 'NONE', #16667, #16437, #20334 ) ;
#5419=CARTESIAN_POINT ( 'NONE',  ( 8.438463404362677167, -11.99816466695113881, 6.398712851742227592 ) ) ;
#5421=EDGE_LOOP ( 'NONE', ( #10520, #14771, #4286, #4710 ) ) ;
#5427=CARTESIAN_POINT ( 'NONE',  ( 7.000000000000006217, -0.9711575687493152476, 9.522727272727294690 ) ) ;
#5440=VERTEX_POINT ( 'NONE', #6994 ) ;
#5446=CARTESIAN_POINT ( 'NONE',  ( 7.271441198316225041, -0.2709289393878955843, 8.039702399269760491 ) ) ;
#5449=CARTESIAN_POINT ( 'NONE',  ( 12.84999999999997300, -1.999999999999998224, 0.000000000000000000 ) ) ;
#5456=DIRECTION ( 'NONE',  ( -1.000000000000000000, -6.224605580259554159E-31, 2.887593071917436153E-31 ) ) ;
#5459=CARTESIAN_POINT ( 'NONE',  ( 7.282868595548843693, -0.2617430505219933701, 8.010178330700751914 ) ) ;
#5465=VERTEX_POINT ( 'NONE', #8740 ) ;
#5466=EDGE_LOOP ( 'NONE', ( #19541, #5133, #6353, #22188 ) ) ;
#5488=CARTESIAN_POINT ( 'NONE',  ( 12.84999999999997300, -12.00000000000011191, -5.749999999999936051 ) ) ;
#5491=EDGE_CURVE ( 'NONE', #5891, #396, #1593, .T. ) ;
#5493=VERTEX_POINT ( 'NONE', #21575 ) ;
#5500=ADVANCED_FACE ( 'NONE', ( #7445 ), #17918, .T. ) ;
#5501=LINE ( 'NONE', #3163, #12872 ) ;
#5506=CARTESIAN_POINT ( 'NONE',  ( -7.132286784435623694, -13.57635026841689019, 8.470912490188640120 ) ) ;
#5516=ADVANCED_FACE ( 'NONE', ( #14499 ), #5221, .F. ) ;
#5521=ORIENTED_EDGE ( 'NONE', *, *, #9147, .T. ) ;
#5527=CARTESIAN_POINT ( 'NONE',  ( 7.162073728446673115, -11.63471678239051954, 7.945145523438290169 ) ) ;
#5531=ORIENTED_EDGE ( 'NONE', *, *, #11979, .F. ) ;
#5533=DIRECTION ( 'NONE',  ( -5.551115123125818447E-17, -6.982962677686276177E-15, -1.000000000000000000 ) ) ;
#5535=CARTESIAN_POINT ( 'NONE',  ( 8.697224362267997222, -14.00000000000004974, 6.250000000000033751 ) ) ;
#5555=CARTESIAN_POINT ( 'NONE',  ( 7.521298409251910400, -11.75792766829873237, 8.817899680514896588 ) ) ;
#5556=CARTESIAN_POINT ( 'NONE',  ( -8.079084010241061264, -11.97965595983265530, 6.665520415301771529 ) ) ;
#5567=DIRECTION ( 'NONE',  ( -1.454462294001240516E-30, -1.000000000000000000, -0.000000000000000000 ) ) ;
#5572=CARTESIAN_POINT ( 'NONE',  ( 7.920269128372694922, -0.6322607639407502589, 7.713069291591495791 ) ) ;
#5597=CARTESIAN_POINT ( 'NONE',  ( -12.84999999999999964, -12.50000000000011191, -5.749999999999936051 ) ) ;
#5623=CARTESIAN_POINT ( 'NONE',  ( 8.113551354210024158, -12.41661007101923531, 7.426820295479682699 ) ) ;
#5628=CARTESIAN_POINT ( 'NONE',  ( 7.955953741309973459, -1.644172503818053688, 7.654083333123856470 ) ) ;
#5634=EDGE_CURVE ( 'NONE', #9332, #10367, #6025, .T. ) ;
#5654=CARTESIAN_POINT ( 'NONE',  ( 7.282868595548778856, -13.73825694947798937, 8.010178330700917115 ) ) ;
#5673=FACE_OUTER_BOUND ( 'NONE', #14310, .T. ) ;
#5686=CARTESIAN_POINT ( 'NONE',  ( 7.576750937466539604, -2.112750738699229469, 7.200086239788012321 ) ) ;
#5698=VERTEX_POINT ( 'NONE', #22722 ) ;
#5699=EDGE_LOOP ( 'NONE', ( #7457, #7370, #9568, #11366 ) ) ;
#5702=DIRECTION ( 'NONE',  ( 0.000000000000000000, 0.000000000000000000, 1.000000000000000000 ) ) ;
#5708=EDGE_CURVE ( 'NONE', #9220, #6218, #1074, .T. ) ;
#5710=CARTESIAN_POINT ( 'NONE',  ( 7.500000000000007105, -8.000000000000017764, 10.24999999999999467 ) ) ;
#5725=TOROIDAL_SURFACE ( 'NONE', #458, 4.500000000000000888, 0.5000000000000000000 ) ;
#5730=CARTESIAN_POINT ( 'NONE',  ( -12.85000000000001386, 0.000000000000000000, -5.749999999999991118 ) ) ;
#5735=DIRECTION ( 'NONE',  ( 0.000000000000000000, 0.000000000000000000, 1.000000000000000000 ) ) ;
#5736=CARTESIAN_POINT ( 'NONE',  ( 7.629227790279509591, -12.04719844907615744, 8.369856247450654152 ) ) ;
#5738=CARTESIAN_POINT ( 'NONE',  ( -7.491585531133505782, -2.143791077336254958, 7.320610673787135703 ) ) ;
#5747=AXIS2_PLACEMENT_3D ( 'NONE', #1499, #22917, #6789 ) ;
#5750=ORIENTED_EDGE ( 'NONE', *, *, #2789, .F. ) ;
#5759=CARTESIAN_POINT ( 'NONE',  ( 7.026577802269679651, -11.35109376985338869, 8.453373545151615431 ) ) ;
#5763=CARTESIAN_POINT ( 'NONE',  ( 12.84999999999998721, -12.50000000000011191, -6.249999999999936051 ) ) ;
#5773=CIRCLE ( 'NONE', #13660, 0.4999999999999995559 ) ;
#5784=EDGE_CURVE ( 'NONE', #10359, #22613, #2566, .T. ) ;
#5789=AXIS2_PLACEMENT_3D ( 'NONE', #11138, #331, #16763 ) ;
#5809=DIRECTION ( 'NONE',  ( 9.121204216617949000E-31, 1.000000000000000000, -6.982962677686261977E-15 ) ) ;
#5812=ORIENTED_EDGE ( 'NONE', *, *, #19181, .T. ) ;
#5822=ORIENTED_EDGE ( 'NONE', *, *, #597, .F. ) ;
#5826=CARTESIAN_POINT ( 'NONE',  ( 12.84999999999997300, -0.5000000000000004441, 1.387778780781445676E-14 ) ) ;
#5832=CARTESIAN_POINT ( 'NONE',  ( -7.161440864725758360, -2.387752514309356311, 7.973376427817367329 ) ) ;
#5850=ORIENTED_EDGE ( 'NONE', *, *, #915, .T. ) ;
#5859=CARTESIAN_POINT ( 'NONE',  ( 12.84999999999997300, -2.011595308313580664E-30, 2.550000000000010925 ) ) ;
#5860=CARTESIAN_POINT ( 'NONE',  ( -12.85000000000001386, -1.999999999999998224, -6.249999999999992006 ) ) ;
#5861=CARTESIAN_POINT ( 'NONE',  ( -12.85000000000002807, -12.00000000000002842, 6.250000000000019540 ) ) ;
#5862=EDGE_CURVE ( 'NONE', #19457, #1155, #18720, .T. ) ;
#5864=CIRCLE ( 'NONE', #19007, 0.5000000000000005551 ) ;
#5869=DIRECTION ( 'NONE',  ( -9.121204216617949000E-31, -1.000000000000000000, 6.982962677686261977E-15 ) ) ;
#5881=CARTESIAN_POINT ( 'NONE',  ( 7.568268608011931242, -13.53268520232752614, 8.579161250779895553 ) ) ;
#5886=CARTESIAN_POINT ( 'NONE',  ( -7.000000000000006217, 2.775557561562891351E-14, 12.24999999999996980 ) ) ;
#5891=VERTEX_POINT ( 'NONE', #23083 ) ;
#5893=CARTESIAN_POINT ( 'NONE',  ( 7.168696526429609861, -0.3737769141893478864, 8.340670630249134021 ) ) ;
#5902=AXIS2_PLACEMENT_3D ( 'NONE', #6618, #6508, #10495 ) ;
#5909=CARTESIAN_POINT ( 'NONE',  ( -12.85000000000001386, -12.00000000000005151, 2.550000000000038902 ) ) ;
#5911=CARTESIAN_POINT ( 'NONE',  ( 8.233775472210654200, -0.5437072270125227202, 7.279685395985851848 ) ) ;
#5917=EDGE_LOOP ( 'NONE', ( #19977, #16108, #13089, #7233 ) ) ;
#5947=CIRCLE ( 'NONE', #5188, 2.549999999999997158 ) ;
#5955=VECTOR ( 'NONE', #15870, 1000.000000000000000 ) ;
#5957=ORIENTED_EDGE ( 'NONE', *, *, #21358, .T. ) ;
#5962=CARTESIAN_POINT ( 'NONE',  ( -12.85000000000001386, -14.00000000000008882, -2.549999999999945199 ) ) ;
#5966=PLANE ( 'NONE',  #21121 ) ;
#5969=DIRECTION ( 'NONE',  ( 0.000000000000000000, 0.000000000000000000, 1.000000000000000000 ) ) ;
#5977=DIRECTION ( 'NONE',  ( -1.000000000000000000, -1.910522504832140594E-31, 5.551115123125818447E-17 ) ) ;
#5992=DIRECTION ( 'NONE',  ( 1.454462294001240516E-30, 1.000000000000000000, 0.000000000000000000 ) ) ;
#5994=DIRECTION ( 'NONE',  ( 1.734723475976813750E-16, 1.000000000000000000, -3.469446951953607484E-15 ) ) ;
#6001=CARTESIAN_POINT ( 'NONE',  ( 7.756475484083226846, -13.93440482874969533, 7.145789564688786122 ) ) ;
#6012=ORIENTED_EDGE ( 'NONE', *, *, #20906, .F. ) ;
#6025=LINE ( 'NONE', #9436, #10988 ) ;
#6027=LINE ( 'NONE', #2485, #22703 ) ;
#6028=DIRECTION ( 'NONE',  ( 0.000000000000000000, -6.938893903907238633E-15, -1.000000000000000000 ) ) ;
#6030=DIRECTION ( 'NONE',  ( -4.019602852144232182E-47, -6.982962677686261977E-15, -1.000000000000000000 ) ) ;
#6031=ORIENTED_EDGE ( 'NONE', *, *, #6805, .F. ) ;
#6039=VERTEX_POINT ( 'NONE', #7874 ) ;
#6075=CYLINDRICAL_SURFACE ( 'NONE', #8996, 2.549999999999997158 ) ;
#6077=CARTESIAN_POINT ( 'NONE',  ( -7.521298409251902406, -11.75792766829873415, 8.817899680514910798 ) ) ;
#6087=AXIS2_PLACEMENT_3D ( 'NONE', #10530, #14182, #3899 ) ;
#6090=EDGE_CURVE ( 'NONE', #195, #10367, #1171, .T. ) ;
#6091=VERTEX_POINT ( 'NONE', #4805 ) ;
#6096=DIRECTION ( 'NONE',  ( 1.000000000000000000, 1.910522504832140594E-31, -5.551115123125818447E-17 ) ) ;
#6099=AXIS2_PLACEMENT_3D ( 'NONE', #1686, #14152, #7332 ) ;
#6111=CARTESIAN_POINT ( 'NONE',  ( -7.733764002503129120, -0.7473006511613556890, 8.082002268151461166 ) ) ;
#6112=CARTESIAN_POINT ( 'NONE',  ( 7.876571740167124247, -13.80606002021554701, 7.785394814391048079 ) ) ;
#6116=( NAMED_UNIT ( * ) PLANE_ANGLE_UNIT ( ) SI_UNIT ( $, .RADIAN. ) );
#6137=DIRECTION ( 'NONE',  ( 1.431475090352998897E-31, -3.469446951953609061E-15, -1.000000000000000000 ) ) ;
#6162=DIRECTION ( 'NONE',  ( 1.454462294001240516E-30, 1.000000000000000000, 0.000000000000000000 ) ) ;
#6171=CARTESIAN_POINT ( 'NONE',  ( -7.499999999999992895, -2.645898033750305522, 9.250000000000014211 ) ) ;
#6174=CARTESIAN_POINT ( 'NONE',  ( 7.710998176012537897, -2.456120859166848192, 8.114728912742497968 ) ) ;
#6181=FACE_OUTER_BOUND ( 'NONE', #21920, .T. ) ;
#6191=AXIS2_PLACEMENT_3D ( 'NONE', #18347, #14689, #4207 ) ;
#6198=CARTESIAN_POINT ( 'NONE',  ( -10.49999999999998224, -12.50000000000000711, 9.250000000000063949 ) ) ;
#6200=CARTESIAN_POINT ( 'NONE',  ( -7.778057173929672885, -12.23790148979555070, 7.981635986975519792 ) ) ;
#6201=CARTESIAN_POINT ( 'NONE',  ( -8.697224362268007880, -14.00000000000004619, 6.250000000000031086 ) ) ;
#6202=DIRECTION ( 'NONE',  ( -1.000000000000000000, -4.252453317207022894E-31, 5.551115123125818447E-17 ) ) ;
#6218=VERTEX_POINT ( 'NONE', #4695 ) ;
#6219=DIRECTION ( 'NONE',  ( 0.000000000000000000, 0.000000000000000000, -1.000000000000000000 ) ) ;
#6222=EDGE_CURVE ( 'NONE', #12422, #22613, #19049, .T. ) ;
#6240=EDGE_CURVE ( 'NONE', #13412, #9370, #9291, .T. ) ;
#6244=CIRCLE ( 'NONE', #3244, 0.4999999999999995559 ) ;
#6262=CARTESIAN_POINT ( 'NONE',  ( -7.000000000000020428, -3.018576030000264865, 8.916666666666712260 ) ) ;
#6280=CARTESIAN_POINT ( 'NONE',  ( -7.778057173929718182, -1.762098510204431756, 7.981635986975294195 ) ) ;
#6283=AXIS2_PLACEMENT_3D ( 'NONE', #13778, #20727, #1089 ) ;
#6286=CARTESIAN_POINT ( 'NONE',  ( 7.854293383767891434, -2.312270958411924315, 7.820081954007007674 ) ) ;
#6292=FACE_OUTER_BOUND ( 'NONE', #5421, .T. ) ;
#6314=AXIS2_PLACEMENT_3D ( 'NONE', #1846, #9034, #12557 ) ;
#6315=CARTESIAN_POINT ( 'NONE',  ( 10.50000000000000888, -12.50000000000002842, 5.750000000000088818 ) ) ;
#6325=AXIS2_PLACEMENT_3D ( 'NONE', #1316, #8484, #4939 ) ;
#6336=CARTESIAN_POINT ( 'NONE',  ( -7.500000000000020428, -6.999999999999995559, 12.24999999999999645 ) ) ;
#6337=DIRECTION ( 'NONE',  ( -4.019602852144215652E-47, -6.982962677686261977E-15, -1.000000000000000000 ) ) ;
#6339=AXIS2_PLACEMENT_3D ( 'NONE', #1400, #15624, #15738 ) ;
#6346=CARTESIAN_POINT ( 'NONE',  ( 8.725359747074524108, -13.50000000719894366, 6.816426071237588147 ) ) ;
#6347=DIRECTION ( 'NONE',  ( 2.168404344971017743E-16, 1.000000000000000000, -6.982962677686261977E-15 ) ) ;
#6351=DIRECTION ( 'NONE',  ( 9.121204216617949000E-31, 1.000000000000000000, -6.982962677686261977E-15 ) ) ;
#6353=ORIENTED_EDGE ( 'NONE', *, *, #2212, .F. ) ;
#6359=ORIENTED_EDGE ( 'NONE', *, *, #8983, .T. ) ;
#6363=DIRECTION ( 'NONE',  ( -0.8571428571428572063, 6.547888496751957777E-15, 0.5150787536377126052 ) ) ;
#6374=PLANE ( 'NONE',  #19987 ) ;
#6395=ADVANCED_FACE ( 'NONE', ( #6292 ), #21385, .T. ) ;
#6404=CARTESIAN_POINT ( 'NONE',  ( 7.120027569165277903, -2.450222941140161037, 8.099087005775102099 ) ) ;
#6420=ADVANCED_FACE ( 'NONE', ( #2638 ), #20647, .T. ) ;
#6429=VECTOR ( 'NONE', #2952, 1000.000000000000000 ) ;
#6431=CARTESIAN_POINT ( 'NONE',  ( -7.467942433933816737, -11.84606835491527121, 7.356484134531112495 ) ) ;
#6432=CARTESIAN_POINT ( 'NONE',  ( -7.573440241539870499, -13.88616620752087982, 7.421600184846463222 ) ) ;
#6439=ORIENTED_EDGE ( 'NONE', *, *, #21749, .T. ) ;
#6446=PLANE ( 'NONE',  #23025 ) ;
#6451=CARTESIAN_POINT ( 'NONE',  ( 12.84999999999997300, -12.00000000000002842, 6.250000000000019540 ) ) ;
#6457=DIRECTION ( 'NONE',  ( 1.000000000000000000, 3.469446951953617344E-15, 0.000000000000000000 ) ) ;
#6458=CIRCLE ( 'NONE', #15825, 0.4999999999999995559 ) ;
#6460=LINE ( 'NONE', #20934, #15526 ) ;
#6481=FACE_OUTER_BOUND ( 'NONE', #4992, .T. ) ;
#6507=VECTOR ( 'NONE', #3069, 1000.000000000000000 ) ;
#6508=DIRECTION ( 'NONE',  ( 9.121204216617949000E-31, 1.000000000000000000, -6.982962677686261977E-15 ) ) ;
#6516=CARTESIAN_POINT ( 'NONE',  ( 7.734741761309861907, -2.069990213851688132, 7.004299047562906111 ) ) ;
#6523=CARTESIAN_POINT ( 'NONE',  ( -1.387778780781445676E-14, 2.775557561562891351E-14, 12.24999999999996980 ) ) ;
#6534=CIRCLE ( 'NONE', #3144, 0.4999999999999987232 ) ;
#6535=EDGE_CURVE ( 'NONE', #6091, #8927, #14554, .T. ) ;
#6541=EDGE_CURVE ( 'NONE', #22613, #13556, #15107, .T. ) ;
#6543=ORIENTED_EDGE ( 'NONE', *, *, #8373, .F. ) ;
#6560=DIRECTION ( 'NONE',  ( -0.5150787536377134934, 0.000000000000000000, -0.8571428571428567622 ) ) ;
#6562=ORIENTED_EDGE ( 'NONE', *, *, #9580, .F. ) ;
#6563=AXIS2_PLACEMENT_3D ( 'NONE', #19682, #3444, #14148 ) ;
#6578=CARTESIAN_POINT ( 'NONE',  ( -7.568268608011889498, -0.4673147976723305286, 8.579161250779817394 ) ) ;
#6581=AXIS2_PLACEMENT_3D ( 'NONE', #9895, #21071, #22837 ) ;
#6587=DIRECTION ( 'NONE',  ( 1.454462294001240516E-30, 1.000000000000000000, 0.000000000000000000 ) ) ;
#6605=CARTESIAN_POINT ( 'NONE',  ( -7.000000000000006217, -5.999999999999987566, 10.24999999999998224 ) ) ;
#6618=CARTESIAN_POINT ( 'NONE',  ( -10.49999999999998224, -12.50000000000000711, 9.250000000000063949 ) ) ;
#6624=EDGE_CURVE ( 'NONE', #7917, #19419, #13823, .T. ) ;
#6632=ADVANCED_FACE ( 'NONE', ( #1902 ), #51, .T. ) ;
#6633=VERTEX_POINT ( 'NONE', #19920 ) ;
#6646=ADVANCED_FACE ( 'NONE', ( #3788 ), #17183, .T. ) ;
#6647=AXIS2_PLACEMENT_3D ( 'NONE', #11303, #5567, #9207 ) ;
#6652=DIRECTION ( 'NONE',  ( 1.000000000000000000, -2.168404344971005170E-16, 1.203141491611682442E-30 ) ) ;
#6672=VECTOR ( 'NONE', #13696, 1000.000000000000000 ) ;
#6674=DIRECTION ( 'NONE',  ( 0.000000000000000000, 0.000000000000000000, -1.000000000000000000 ) ) ;
#6681=DIRECTION ( 'NONE',  ( -9.121204216617949000E-31, -1.000000000000000000, 6.982962677686261977E-15 ) ) ;
#6687=CARTESIAN_POINT ( 'NONE',  ( -8.954763739086818219, -0.4999999999999885092, 6.678571428571394186 ) ) ;
#6688=VECTOR ( 'NONE', #8654, 1000.000000000000000 ) ;
#6698=EDGE_CURVE ( 'NONE', #11731, #11726, #7779, .T. ) ;
#6699=DIRECTION ( 'NONE',  ( 1.454462294001240516E-30, 1.000000000000000000, 0.000000000000000000 ) ) ;
#6709=CARTESIAN_POINT ( 'NONE',  ( -12.85000000000004228, -0.5000000000000004441, -6.249999999999977796 ) ) ;
#6714=FACE_OUTER_BOUND ( 'NONE', #4026, .T. ) ;
#6722=CIRCLE ( 'NONE', #15728, 0.4999999999999990563 ) ;
#6724=VERTEX_POINT ( 'NONE', #17059 ) ;
#6727=VERTEX_POINT ( 'NONE', #11425 ) ;
#6733=CARTESIAN_POINT ( 'NONE',  ( 12.84999999999997300, -1.500000000000001332, 6.250000000000005329 ) ) ;
#6737=CARTESIAN_POINT ( 'NONE',  ( -7.000000000000006217, -0.9711575687493188003, 9.522727272727280479 ) ) ;
#6738=CARTESIAN_POINT ( 'NONE',  ( -8.181569977154534712, -2.135203747983297262, 7.340676138759476110 ) ) ;
#6745=EDGE_CURVE ( 'NONE', #20589, #18641, #15669, .T. ) ;
#6775=B_SPLINE_CURVE_WITH_KNOTS ( 'NONE', 3,
 ( #12691, #7179, #5759, #5527, #21535, #14339, #16328, #11037, #16439, #19760, #2219, #5419, #1978, #21649 ),
 .UNSPECIFIED., .F., .F.,
 ( 4, 2, 2, 2, 2, 2, 4 ),
 ( 0.000000000000000000, 0.0008860460682957670793, 0.001772092136591534159, 0.002215115170739416234, 0.002658138204887298961, 0.003101161239035180820, 0.003544184273183063547 ),
 .UNSPECIFIED. ) ;
#6777=CARTESIAN_POINT ( 'NONE',  ( 8.200527591913237657, -12.43937801162580925, 7.318116290495840559 ) ) ;
#6787=ORIENTED_EDGE ( 'NONE', *, *, #1501, .F. ) ;
#6788=ORIENTED_EDGE ( 'NONE', *, *, #20906, .T. ) ;
#6789=DIRECTION ( 'NONE',  ( -1.000000000000000000, -3.469446951953617344E-15, 0.000000000000000000 ) ) ;
#6792=CARTESIAN_POINT ( 'NONE',  ( -12.84999999999999964, -14.00000000000003020, 5.750000000000032863 ) ) ;
#6805=EDGE_CURVE ( 'NONE', #9710, #11691, #16424, .T. ) ;
#6807=EDGE_CURVE ( 'NONE', #18911, #9721, #18487, .T. ) ;
#6808=EDGE_CURVE ( 'NONE', #14530, #9714, #16058, .T. ) ;
#6817=ORIENTED_EDGE ( 'NONE', *, *, #4481, .F. ) ;
#6819=CARTESIAN_POINT ( 'NONE',  ( -7.499999999999992895, -5.999999999999981348, 11.74999999999998224 ) ) ;
#6821=CYLINDRICAL_SURFACE ( 'NONE', #9985, 2.999999999999995559 ) ;
#6824=EDGE_CURVE ( 'NONE', #20968, #17687, #11928, .T. ) ;
#6830=DIRECTION ( 'NONE',  ( -1.000000000000000000, -4.252453317207022018E-31, 5.551115123125818447E-17 ) ) ;
#6834=CARTESIAN_POINT ( 'NONE',  ( -7.000000000000033751, -11.35410196624970780, 9.250000000000063949 ) ) ;
#6839=ORIENTED_EDGE ( 'NONE', *, *, #7772, .F. ) ;
#6850=CARTESIAN_POINT ( 'NONE',  ( -12.85000000000002807, -12.00000000000002842, 6.250000000000019540 ) ) ;
#6854=FACE_OUTER_BOUND ( 'NONE', #5343, .T. ) ;
#6861=DIRECTION ( 'NONE',  ( -1.232595164407830946E-32, 1.000000000000000000, -6.938893903907214967E-15 ) ) ;
#6866=CARTESIAN_POINT ( 'NONE',  ( -7.629227790279501598, -12.04719844907614146, 8.369856247450657705 ) ) ;
#6891=CARTESIAN_POINT ( 'NONE',  ( -7.523653856849436217, -1.079621694564730783, 8.801128846369456582 ) ) ;
#6925=DIRECTION ( 'NONE',  ( -9.121204216617949000E-31, -1.000000000000000000, 6.982962677686261977E-15 ) ) ;
#6926=CARTESIAN_POINT ( 'NONE',  ( -7.951003271401643424, -0.1617022081437910763, 7.659883344695618490 ) ) ;
#6930=DIRECTION ( 'NONE',  ( 0.000000000000000000, 0.000000000000000000, -1.000000000000000000 ) ) ;
#6931=DIRECTION ( 'NONE',  ( 0.000000000000000000, 0.000000000000000000, -1.000000000000000000 ) ) ;
#6936=AXIS2_PLACEMENT_3D ( 'NONE', #967, #4588, #4938 ) ;
#6938=VERTEX_POINT ( 'NONE', #6605 ) ;
#6957=EDGE_CURVE ( 'NONE', #8927, #4863, #20961, .T. ) ;
#6960=CARTESIAN_POINT ( 'NONE',  ( -8.414481090081503467, -14.00000000000004263, 6.435353702847475432 ) ) ;
#6962=CARTESIAN_POINT ( 'NONE',  ( 7.500000000000007105, -2.645898033750298417, 9.250000000000019540 ) ) ;
#6975=ORIENTED_EDGE ( 'NONE', *, *, #1042, .T. ) ;
#6986=CARTESIAN_POINT ( 'NONE',  ( -8.195710046796570225, -11.98804095514285351, 6.570882465138064177 ) ) ;
#6989=CARTESIAN_POINT ( 'NONE',  ( 12.84999999999997300, 0.000000000000000000, -5.749999999999976907 ) ) ;
#6994=CARTESIAN_POINT ( 'NONE',  ( -12.84999999999999964, -14.00000000000011369, -5.749999999999949374 ) ) ;
#7018=CARTESIAN_POINT ( 'NONE',  ( -6.999999999999992006, -13.02884243125069652, 9.522727272727321335 ) ) ;
#7029=ORIENTED_EDGE ( 'NONE', *, *, #21335, .F. ) ;
#7030=VERTEX_POINT ( 'NONE', #10709 ) ;
#7033=CIRCLE ( 'NONE', #6647, 3.499999999999996003 ) ;
#7045=AXIS2_PLACEMENT_3D ( 'NONE', #2715, #9668, #13322 ) ;
#7060=CYLINDRICAL_SURFACE ( 'NONE', #21568, 6.249999999999992006 ) ;
#7062=EDGE_LOOP ( 'NONE', ( #8703, #7943, #8170, #7456 ) ) ;
#7064=LINE ( 'NONE', #23067, #17410 ) ;
#7076=EDGE_CURVE ( 'NONE', #3180, #16622, #12711, .T. ) ;
#7083=CIRCLE ( 'NONE', #21359, 0.4999999999999998335 ) ;
#7104=DIRECTION ( 'NONE',  ( 1.454462294001240516E-30, 1.000000000000000000, 0.000000000000000000 ) ) ;
#7109=EDGE_CURVE ( 'NONE', #5493, #9975, #1540, .T. ) ;
#7114=CARTESIAN_POINT ( 'NONE',  ( 12.84999999999997300, -12.50000000000002842, 5.750000000000088818 ) ) ;
#7120=ORIENTED_EDGE ( 'NONE', *, *, #2212, .T. ) ;
#7122=ORIENTED_EDGE ( 'NONE', *, *, #22740, .T. ) ;
#7135=CARTESIAN_POINT ( 'NONE',  ( -7.523653856849478849, -12.92037830543528010, 8.801128846369513425 ) ) ;
#7139=CARTESIAN_POINT ( 'NONE',  ( 7.499999999999992895, -5.999999999999981348, 6.250000000000005329 ) ) ;
#7143=DIRECTION ( 'NONE',  ( 0.000000000000000000, 0.000000000000000000, 1.000000000000000000 ) ) ;
#7149=VECTOR ( 'NONE', #5994, 1000.000000000000000 ) ;
#7159=DIRECTION ( 'NONE',  ( 0.000000000000000000, 6.802837160693368935E-15, 1.000000000000000000 ) ) ;
#7162=CARTESIAN_POINT ( 'NONE',  ( 7.500000000000007105, -8.000000000000003553, 12.24999999999999645 ) ) ;
#7164=CARTESIAN_POINT ( 'NONE',  ( -6.999999999999978684, 2.428612866367529932E-14, 11.74999999999996803 ) ) ;
#7170=DIRECTION ( 'NONE',  ( 1.000000000000000000, 6.224605580259554159E-31, -2.887593071917436153E-31 ) ) ;
#7171=CARTESIAN_POINT ( 'NONE',  ( -10.49999999999998224, -13.50000000000003020, 6.250000000000033751 ) ) ;
#7177=DIRECTION ( 'NONE',  ( 0.000000000000000000, -7.888609052210128564E-31, 1.000000000000000000 ) ) ;
#7179=CARTESIAN_POINT ( 'NONE',  ( 6.999999999999977796, -11.18103031733298458, 8.693499985977936717 ) ) ;
#7180=EDGE_CURVE ( 'NONE', #7803, #6727, #16562, .T. ) ;
#7198=ORIENTED_EDGE ( 'NONE', *, *, #22611, .F. ) ;
#7202=AXIS2_PLACEMENT_3D ( 'NONE', #11619, #17025, #11500 ) ;
#7226=EDGE_LOOP ( 'NONE', ( #828, #7029, #3454, #13204 ) ) ;
#7231=AXIS2_PLACEMENT_3D ( 'NONE', #18633, #4271, #21946 ) ;
#7233=ORIENTED_EDGE ( 'NONE', *, *, #6824, .F. ) ;
#7239=CARTESIAN_POINT ( 'NONE',  ( -8.954763739086866181, -13.50000000000003553, 6.678571428571478563 ) ) ;
#7245=DIRECTION ( 'NONE',  ( 1.000000000000000000, 2.168404344971017743E-16, -1.780660105995169760E-30 ) ) ;
#7266=EDGE_CURVE ( 'NONE', #3149, #16593, #15340, .T. ) ;
#7270=EDGE_CURVE ( 'NONE', #21059, #9302, #2820, .T. ) ;
#7271=CARTESIAN_POINT ( 'NONE',  ( 12.84999999999997300, -14.00000000000007105, 5.551115123125782702E-14 ) ) ;
#7280=CARTESIAN_POINT ( 'NONE',  ( -7.000000000000020428, -2.818969682667033183, 8.693499985977942046 ) ) ;
#7283=DIRECTION ( 'NONE',  ( 2.168404344971017743E-16, 1.000000000000000000, -6.982962677686261977E-15 ) ) ;
#7286=FACE_OUTER_BOUND ( 'NONE', #12453, .T. ) ;
#7289=CIRCLE ( 'NONE', #15527, 0.4999999999999987232 ) ;
#7294=EDGE_CURVE ( 'NONE', #19001, #3406, #6722, .T. ) ;
#7304=EDGE_CURVE ( 'NONE', #10857, #8955, #13473, .T. ) ;
#7316=ORIENTED_EDGE ( 'NONE', *, *, #19074, .T. ) ;
#7325=CARTESIAN_POINT ( 'NONE',  ( 8.414481090081473269, 1.737226928909803488E-14, 6.435353702847417701 ) ) ;
#7332=DIRECTION ( 'NONE',  ( 0.000000000000000000, -6.938893903907237055E-15, -1.000000000000000000 ) ) ;
#7339=ORIENTED_EDGE ( 'NONE', *, *, #11419, .T. ) ;
#7349=ORIENTED_EDGE ( 'NONE', *, *, #2620, .T. ) ;
#7359=EDGE_CURVE ( 'NONE', #20629, #20539, #16842, .T. ) ;
#7362=DIRECTION ( 'NONE',  ( 1.000000000000000000, 2.168404344970994323E-16, -1.780660105995169760E-30 ) ) ;
#7370=ORIENTED_EDGE ( 'NONE', *, *, #18745, .F. ) ;
#7371=EDGE_CURVE ( 'NONE', #6724, #4343, #2198, .T. ) ;
#7372=EDGE_LOOP ( 'NONE', ( #21559, #13622, #13620, #18767, #18201, #12948, #18388, #20658 ) ) ;
#7387=LINE ( 'NONE', #21850, #14794 ) ;
#7401=CARTESIAN_POINT ( 'NONE',  ( -12.84999999999999964, -1.499999999999997780, 6.250000000000033751 ) ) ;
#7412=CARTESIAN_POINT ( 'NONE',  ( 8.429621201838076061, -14.00000000000004974, 6.425428529986020543 ) ) ;
#7416=SURFACE_SIDE_STYLE ('',( #18352 ) ) ;
#7420=AXIS2_PLACEMENT_3D ( 'NONE', #224, #19513, #10455 ) ;
#7427=ORIENTED_EDGE ( 'NONE', *, *, #14825, .F. ) ;
#7432=CARTESIAN_POINT ( 'NONE',  ( 7.778057173929708412, -12.23790148979555070, 7.981635986975476271 ) ) ;
#7435=CIRCLE ( 'NONE', #21355, 0.4999999999999995559 ) ;
#7436=DIRECTION ( 'NONE',  ( 1.000000000000000000, 4.252453317207022018E-31, -5.551115123125818447E-17 ) ) ;
#7445=FACE_OUTER_BOUND ( 'NONE', #21060, .T. ) ;
#7448=CARTESIAN_POINT ( 'NONE',  ( -12.84999999999999964, -1.500000000000001332, 0.000000000000000000 ) ) ;
#7456=ORIENTED_EDGE ( 'NONE', *, *, #21108, .T. ) ;
#7457=ORIENTED_EDGE ( 'NONE', *, *, #5389, .T. ) ;
#7492=AXIS2_PLACEMENT_3D ( 'NONE', #14267, #19681, #9200 ) ;
#7497=CARTESIAN_POINT ( 'NONE',  ( -7.499999999999988454, -12.78258024831861661, 9.022398393215850021 ) ) ;
#7504=DIRECTION ( 'NONE',  ( -1.000000000000000000, 2.168404344971005170E-16, -1.203141491611682442E-30 ) ) ;
#7515=AXIS2_PLACEMENT_3D ( 'NONE', #13932, #10526, #12515 ) ;
#7527=CARTESIAN_POINT ( 'NONE',  ( 8.148407558030035247, -13.43987109532831070, 7.382406087064103950 ) ) ;
#7541=ORIENTED_EDGE ( 'NONE', *, *, #21078, .F. ) ;
#7550=CARTESIAN_POINT ( 'NONE',  ( -12.84999999999999964, -6.938893903907228378E-15, 5.749999999999991118 ) ) ;
#7561=CARTESIAN_POINT ( 'NONE',  ( 7.479729963966237349, -0.8034648269415383126, 9.265052153039572858 ) ) ;
#7580=CARTESIAN_POINT ( 'NONE',  ( -7.024848138040975520, -2.659619850263430507, 8.468562630484278486 ) ) ;
#7584=DIRECTION ( 'NONE',  ( 0.000000000000000000, 0.000000000000000000, 1.000000000000000000 ) ) ;
#7604=CYLINDRICAL_SURFACE ( 'NONE', #3360, 2.549999999999997158 ) ;
#7631=CIRCLE ( 'NONE', #8392, 0.4999999999999999445 ) ;
#7636=DIRECTION ( 'NONE',  ( 0.000000000000000000, 0.000000000000000000, 1.000000000000000000 ) ) ;
#7658=CARTESIAN_POINT ( 'NONE',  ( 7.332081355611481222, -0.2267865287842198430, 7.890992604157067269 ) ) ;
#7660=VECTOR ( 'NONE', #18902, 1000.000000000000000 ) ;
#7665=AXIS2_PLACEMENT_3D ( 'NONE', #807, #11958, #1273 ) ;
#7666=CARTESIAN_POINT ( 'NONE',  ( 7.500000000000007105, -8.000000000000003553, 12.24999999999999645 ) ) ;
#7676=EDGE_CURVE ( 'NONE', #13819, #19925, #13491, .T. ) ;
#7679=CARTESIAN_POINT ( 'NONE',  ( 7.132286784435700078, -0.4236497315830464183, 8.470912490188409194 ) ) ;
#7710=VERTEX_POINT ( 'NONE', #1598 ) ;
#7722=FACE_OUTER_BOUND ( 'NONE', #12118, .T. ) ;
#7726=CARTESIAN_POINT ( 'NONE',  ( 6.999999999999978684, -8.000000000000017764, 10.24999999999998224 ) ) ;
#7747=DIRECTION ( 'NONE',  ( -1.000000000000000000, -1.910522504832140594E-31, 5.551115123125818447E-17 ) ) ;
#7751=AXIS2_PLACEMENT_3D ( 'NONE', #4049, #14756, #19948 ) ;
#7758=TOROIDAL_SURFACE ( 'NONE', #2128, 5.750000000000000000, 0.5000000000000000000 ) ;
#7772=EDGE_CURVE ( 'NONE', #16593, #1206, #21137, .T. ) ;
#7778=CARTESIAN_POINT ( 'NONE',  ( -12.85000000000004228, -1.499999999999997780, -6.249999999999977796 ) ) ;
#7779=B_SPLINE_CURVE_WITH_KNOTS ( 'NONE', 3,
 ( #16366, #268, #11077, #2135, #14616, #3450, #21804, #5686, #10617, #21462, #5331, #17922, #4129, #18382 ),
 .UNSPECIFIED., .F., .F.,
 ( 4, 2, 2, 2, 2, 2, 4 ),
 ( 0.000000000000000000, 0.0004465115319127612543, 0.0008930230638255225086, 0.001339534595738283871, 0.001786046127651045017, 0.002679069191476569911, 0.003572092255302094805 ),
 .UNSPECIFIED. ) ;
#7782=EDGE_CURVE ( 'NONE', #635, #17483, #21400, .T. ) ;
#7783=CARTESIAN_POINT ( 'NONE',  ( 7.499999999999992895, -5.999999999999981348, 6.250000000000005329 ) ) ;
#7784=DIRECTION ( 'NONE',  ( 1.000000000000000000, -2.168404344971005170E-16, 1.203141491611682442E-30 ) ) ;
#7789=ORIENTED_EDGE ( 'NONE', *, *, #8205, .F. ) ;
#7799=ORIENTED_EDGE ( 'NONE', *, *, #6807, .T. ) ;
#7800=DIRECTION ( 'NONE',  ( -1.000000000000000000, -2.168404344971017743E-16, 1.780660105995169760E-30 ) ) ;
#7803=VERTEX_POINT ( 'NONE', #5488 ) ;
#7814=DIRECTION ( 'NONE',  ( 0.000000000000000000, -0.8381404052084435730, -0.5454545454545466354 ) ) ;
#7820=EDGE_CURVE ( 'NONE', #22329, #3406, #4847, .T. ) ;
#7827=ORIENTED_EDGE ( 'NONE', *, *, #14716, .F. ) ;
#7831=AXIS2_PLACEMENT_3D ( 'NONE', #6834, #20853, #4479 ) ;
#7846=AXIS2_PLACEMENT_3D ( 'NONE', #9006, #19584, #21602 ) ;
#7847=CARTESIAN_POINT ( 'NONE',  ( 8.954763739086851970, -1.500000000000001332, 6.678571428571422608 ) ) ;
#7854=MECHANICAL_DESIGN_GEOMETRIC_PRESENTATION_REPRESENTATION('',(#12342),#2208);
#7871=CARTESIAN_POINT ( 'NONE',  ( 7.573440241539870499, -13.88616620752088160, 7.421600184846474768 ) ) ;
#7874=CARTESIAN_POINT ( 'NONE',  ( -12.84999999999999964, -2.000000000000001776, -2.550000000000000711 ) ) ;
#7879=CIRCLE ( 'NONE', #7515, 6.000000000000000000 ) ;
#7885=ORIENTED_EDGE ( 'NONE', *, *, #9831, .T. ) ;
#7890=DIRECTION ( 'NONE',  ( 0.000000000000000000, -0.7453559924999247910, 0.6666666666666722918 ) ) ;
#7894=CARTESIAN_POINT ( 'NONE',  ( -10.49999999999996803, -0.5000000000000004441, 9.250000000000035527 ) ) ;
#7902=CARTESIAN_POINT ( 'NONE',  ( 12.84999999999997300, -12.00000000000008704, -2.549999999999955413 ) ) ;
#7910=ORIENTED_EDGE ( 'NONE', *, *, #21335, .T. ) ;
#7912=ORIENTED_EDGE ( 'NONE', *, *, #13472, .T. ) ;
#7913=CIRCLE ( 'NONE', #791, 0.5000000000000002220 ) ;
#7914=EDGE_LOOP ( 'NONE', ( #2438, #2152, #19133, #2554 ) ) ;
#7917=VERTEX_POINT ( 'NONE', #11335 ) ;
#7930=AXIS2_PLACEMENT_3D ( 'NONE', #3955, #15956, #1619 ) ;
#7933=CYLINDRICAL_SURFACE ( 'NONE', #14169, 3.999999999999994671 ) ;
#7943=ORIENTED_EDGE ( 'NONE', *, *, #14431, .T. ) ;
#7946=VECTOR ( 'NONE', #14807, 1000.000000000000000 ) ;
#7955=CARTESIAN_POINT ( 'NONE',  ( -7.500000000000031974, -11.57130297831456645, 9.041853041249030554 ) ) ;
#7968=EDGE_LOOP ( 'NONE', ( #13507, #406, #3713, #4034, #22538, #3323 ) ) ;
#7983=LINE ( 'NONE', #16674, #1548 ) ;
#7987=AXIS2_PLACEMENT_3D ( 'NONE', #2038, #13955, #6674 ) ;
#7998=ORIENTED_EDGE ( 'NONE', *, *, #6222, .F. ) ;
#8002=ORIENTED_EDGE ( 'NONE', *, *, #15948, .T. ) ;
#8003=ORIENTED_EDGE ( 'NONE', *, *, #9187, .F. ) ;
#8011=CARTESIAN_POINT ( 'NONE',  ( -12.85000000000001386, -12.00000000000008704, -2.549999999999955413 ) ) ;
#8031=ORIENTED_EDGE ( 'NONE', *, *, #14291, .F. ) ;
#8040=CARTESIAN_POINT ( 'NONE',  ( -12.85000000000001386, -12.00000000000006928, 4.163336342344337027E-14 ) ) ;
#8044=CARTESIAN_POINT ( 'NONE',  ( 7.602880770961811585, -2.006500808705091732, 8.461619612152045278 ) ) ;
#8052=AXIS2_PLACEMENT_3D ( 'NONE', #10974, #526, #14862 ) ;
#8057=ORIENTED_EDGE ( 'NONE', *, *, #13570, .F. ) ;
#8060=ORIENTED_EDGE ( 'NONE', *, *, #9103, .F. ) ;
#8066=FACE_BOUND ( 'NONE', #5127, .T. ) ;
#8067=EDGE_CURVE ( 'NONE', #6633, #3351, #12366, .T. ) ;
#8077=VERTEX_POINT ( 'NONE', #6989 ) ;
#8079=ADVANCED_FACE ( 'NONE', ( #12371 ), #19554, .T. ) ;
#8080=SURFACE_STYLE_FILL_AREA ( #3020 ) ;
#8081=CARTESIAN_POINT ( 'NONE',  ( 8.697224362267997222, -13.50000000000004974, 6.250000000000033751 ) ) ;
#8092=DIRECTION ( 'NONE',  ( 1.000000000000000000, 4.252453317207022018E-31, -5.551115123125818447E-17 ) ) ;
#8108=EDGE_CURVE ( 'NONE', #20416, #21919, #18099, .T. ) ;
#8118=AXIS2_PLACEMENT_3D ( 'NONE', #453, #9279, #13275 ) ;
#8120=DIRECTION ( 'NONE',  ( -2.168404344971008868E-16, 1.000000000000000000, -8.023096076392732812E-15 ) ) ;
#8139=DIRECTION ( 'NONE',  ( -1.454462294001240516E-30, -1.000000000000000000, -0.000000000000000000 ) ) ;
#8141=ORIENTED_EDGE ( 'NONE', *, *, #14205, .F. ) ;
#8143=EDGE_LOOP ( 'NONE', ( #2668, #923, #19142, #4060 ) ) ;
#8155=CARTESIAN_POINT ( 'NONE',  ( -8.723547172042966480, -2.015988055643601395, 6.817515300137126921 ) ) ;
#8163=DIRECTION ( 'NONE',  ( -1.000000000000000000, -4.252453317207022018E-31, 5.551115123125818447E-17 ) ) ;
#8170=ORIENTED_EDGE ( 'NONE', *, *, #16090, .F. ) ;
#8177=ORIENTED_EDGE ( 'NONE', *, *, #22600, .F. ) ;
#8188=( BOUNDED_SURFACE ( )  B_SPLINE_SURFACE ( 3, 2, ( 
 ( #6171, #15081, #11098 ),
 ( #9692, #4151, #11563 ),
 ( #760, #20168, #7580 ),
 ( #18400, #9347, #11323 ),
 ( #2159, #21942, #5832 ),
 ( #16735, #14978, #13687 ),
 ( #6280, #9927, #20752 ),
 ( #17077, #20870, #15204 ),
 ( #19090, #2981, #8280 ),
 ( #22861, #6738, #15436 ),
 ( #15555, #22743, #10152 ),
 ( #12017, #8394, #20979 ),
 ( #1112, #8155, #3098 ),
 ( #13455, #20639, #10037 ) ),
 .UNSPECIFIED., .F., .F., .F. ) 
 B_SPLINE_SURFACE_WITH_KNOTS ( ( 4, 2, 2, 2, 2, 2, 4 ),
 ( 3, 3 ),
 ( 0.000000000000000000, 0.0009656398008937970437, 0.001448459701340695620, 0.001931279601787594087, 0.002414099502234492555, 0.002896919402681391240, 0.003862559203575188175 ),
 ( 0.000000000000000000, 1.000000000000000000 ),
 .UNSPECIFIED. ) 
 GEOMETRIC_REPRESENTATION_ITEM ( )  RATIONAL_B_SPLINE_SURFACE ( (
 ( 1.000000000000000000, 0.7071067811865516806, 1.000000000000000000),
 ( 1.000000000000000000, 0.6907538105667505590, 1.000000000000000000),
 ( 1.000000000000000000, 0.6765417438349563550, 1.000000000000000000),
 ( 1.000000000000000000, 0.6623232117678578001, 1.000000000000000000),
 ( 1.000000000000000000, 0.6588386061807489646, 1.000000000000000000),
 ( 1.000000000000000000, 0.6547992448370589802, 1.000000000000000000),
 ( 1.000000000000000000, 0.6542040191408916572, 1.000000000000000000),
 ( 1.000000000000000000, 0.6557724471762208518, 1.000000000000000000),
 ( 1.000000000000000000, 0.6579729115736204781, 1.000000000000000000),
 ( 1.000000000000000000, 0.6644691908066192587, 1.000000000000000000),
 ( 1.000000000000000000, 0.6687559023949275483, 1.000000000000000000),
 ( 1.000000000000000000, 0.6835702420294330617, 1.000000000000000000),
 ( 1.000000000000000000, 0.6960226107070184298, 1.000000000000000000),
 ( 1.000000000000000000, 0.7071067811865491270, 1.000000000000000000) ) ) 
 REPRESENTATION_ITEM ( '' )  SURFACE ( )  );
#8193=CARTESIAN_POINT ( 'NONE',  ( -7.500000000000034639, -11.35410196624970780, 9.250000000000056843 ) ) ;
#8197=DIRECTION ( 'NONE',  ( 2.891205793294678326E-16, 1.000000000000000000, -6.216092455583559018E-15 ) ) ;
#8205=EDGE_CURVE ( 'NONE', #8955, #19419, #9394, .T. ) ;
#8206=EDGE_LOOP ( 'NONE', ( #21980, #15169, #1877, #19698 ) ) ;
#8210=ADVANCED_FACE ( 'NONE', ( #2558 ), #6446, .T. ) ;
#8220=DIRECTION ( 'NONE',  ( -1.000000000000000000, -6.224605580259554159E-31, 2.887593071917436153E-31 ) ) ;
#8223=CARTESIAN_POINT ( 'NONE',  ( -7.176407415341960139, -0.3641807091869828650, 8.314790908397480251 ) ) ;
#8234=EDGE_CURVE ( 'NONE', #10470, #4924, #13504, .T. ) ;
#8253=CARTESIAN_POINT ( 'NONE',  ( -7.000000000000006217, -0.9711575687493188003, 9.522727272727280479 ) ) ;
#8274=CARTESIAN_POINT ( 'NONE',  ( -6.999999999999992006, -5.999999999999987566, 12.24999999999996980 ) ) ;
#8280=CARTESIAN_POINT ( 'NONE',  ( -7.551224464536099745, -2.121331013966575529, 7.234820221745193791 ) ) ;
#8283=CARTESIAN_POINT ( 'NONE',  ( 7.901093513163758075, -1.673173099260845120, 7.745538272134582236 ) ) ;
#8290=ORIENTED_EDGE ( 'NONE', *, *, #4753, .T. ) ;
#8301=VERTEX_POINT ( 'NONE', #10971 ) ;
#8312=CARTESIAN_POINT ( 'NONE',  ( 7.500000000000007105, -1.999999999999991340, 12.24999999999995559 ) ) ;
#8331=CARTESIAN_POINT ( 'NONE',  ( -7.490952241692738767, -0.6544882962156418627, 8.992386117842782411 ) ) ;
#8336=LINE ( 'NONE', #22811, #9141 ) ;
#8340=CARTESIAN_POINT ( 'NONE',  ( 12.84999999999997300, -12.00000000000006928, 4.163336342344337027E-14 ) ) ;
#8352=ADVANCED_BREP_SHAPE_REPRESENTATION ( '', ( #21131, #22115 ), #3350 ) ;
#8358=EDGE_CURVE ( 'NONE', #3180, #5440, #18884, .T. ) ;
#8369=AXIS2_PLACEMENT_3D ( 'NONE', #19143, #8092, #6219 ) ;
#8373=EDGE_CURVE ( 'NONE', #5891, #7803, #13634, .T. ) ;
#8378=UNCERTAINTY_MEASURE_WITH_UNIT (LENGTH_MEASURE( 1.000000000000000082E-05 ), #9637, 'distance_accuracy_value', 'NONE');
#8389=DIRECTION ( 'NONE',  ( 0.000000000000000000, 0.000000000000000000, -1.000000000000000000 ) ) ;
#8392=AXIS2_PLACEMENT_3D ( 'NONE', #13343, #20523, #18857 ) ;
#8394=CARTESIAN_POINT ( 'NONE',  ( -8.518530740350071184, -2.043531002858365309, 6.984205661426909906 ) ) ;
#8411=EDGE_CURVE ( 'NONE', #20776, #11755, #13849, .T. ) ;
#8424=ORIENTED_EDGE ( 'NONE', *, *, #10825, .F. ) ;
#8431=CIRCLE ( 'NONE', #14817, 0.4999999999999987232 ) ;
#8436=EDGE_CURVE ( 'NONE', #6938, #20539, #12119, .T. ) ;
#8441=ORIENTED_EDGE ( 'NONE', *, *, #14485, .T. ) ;
#8442=EDGE_CURVE ( 'NONE', #7710, #14484, #1606, .T. ) ;
#8444=ORIENTED_EDGE ( 'NONE', *, *, #7304, .T. ) ;
#8446=ORIENTED_EDGE ( 'NONE', *, *, #7270, .F. ) ;
#8452=CARTESIAN_POINT ( 'NONE',  ( -12.85000000000005649, -12.00000000000011191, -6.249999999999936051 ) ) ;
#8455=CARTESIAN_POINT ( 'NONE',  ( -7.000000000000020428, -0.9711575687493234632, 9.522727272727296466 ) ) ;
#8479=CARTESIAN_POINT ( 'NONE',  ( 12.84999999999995879, -0.5000000000000004441, 6.250000000000047073 ) ) ;
#8484=DIRECTION ( 'NONE',  ( -1.000000000000000000, -2.168404344971017743E-16, 1.780660105995169760E-30 ) ) ;
#8500=AXIS2_PLACEMENT_3D ( 'NONE', #5122, #12283, #12048 ) ;
#8505=EDGE_CURVE ( 'NONE', #21059, #6039, #4971, .T. ) ;
#8506=PLANE ( 'NONE',  #17388 ) ;
#8512=DIRECTION ( 'NONE',  ( 1.454462294001240516E-30, 1.000000000000000000, 0.000000000000000000 ) ) ;
#8515=DIRECTION ( 'NONE',  ( 1.000000000000000000, 1.910522504832140594E-31, -5.551115123125818447E-17 ) ) ;
#8530=ORIENTED_EDGE ( 'NONE', *, *, #50, .T. ) ;
#8534=ADVANCED_FACE ( 'NONE', ( #20160 ), #403, .F. ) ;
#8539=EDGE_CURVE ( 'NONE', #10463, #3117, #13648, .T. ) ;
#8544=CARTESIAN_POINT ( 'NONE',  ( -7.500000000000008882, -2.439868446130576629, 9.052558787159767917 ) ) ;
#8547=( NAMED_UNIT ( * ) SI_UNIT ( $, .STERADIAN. ) SOLID_ANGLE_UNIT ( ) );
#8548=DIRECTION ( 'NONE',  ( -9.121204216617949000E-31, -1.000000000000000000, 6.982962677686261977E-15 ) ) ;
#8550=EDGE_LOOP ( 'NONE', ( #14631, #21558, #605, #7427 ) ) ;
#8568=CARTESIAN_POINT ( 'NONE',  ( -7.920269128372646072, -0.6322607639407478164, 7.713069291591470034 ) ) ;
#8573=DIRECTION ( 'NONE',  ( -7.216449660063526979E-15, -6.938893903907237055E-15, -1.000000000000000000 ) ) ;
#8574=VECTOR ( 'NONE', #23111, 1000.000000000000000 ) ;
#8592=ADVANCED_FACE ( 'NONE', ( #19199 ), #19658, .T. ) ;
#8618=CARTESIAN_POINT ( 'NONE',  ( 8.502135871254308697, -13.49242826152325314, 6.995667647939222356 ) ) ;
#8626=CARTESIAN_POINT ( 'NONE',  ( -7.500000000000007105, -11.35410196624970780, 9.250000000000035527 ) ) ;
#8634=ORIENTED_EDGE ( 'NONE', *, *, #21078, .T. ) ;
#8641=VERTEX_POINT ( 'NONE', #22855 ) ;
#8654=DIRECTION ( 'NONE',  ( 1.000000000000000000, 2.312964634635752325E-16, -1.880120159248731926E-30 ) ) ;
#8673=CARTESIAN_POINT ( 'NONE',  ( 8.954763739086823549, -0.5000000000000004441, 6.678571428571450141 ) ) ;
#8679=CARTESIAN_POINT ( 'NONE',  ( -8.148407558029997944, -0.5601289046717349285, 7.382406087064004474 ) ) ;
#8689=DIRECTION ( 'NONE',  ( 1.000000000000000000, 2.168404344971017743E-16, -1.780660105995169760E-30 ) ) ;
#8693=ORIENTED_EDGE ( 'NONE', *, *, #22114, .F. ) ;
#8697=CARTESIAN_POINT ( 'NONE',  ( -12.84999999999999964, -2.000000000000001776, 0.000000000000000000 ) ) ;
#8698=ORIENTED_EDGE ( 'NONE', *, *, #3989, .F. ) ;
#8703=ORIENTED_EDGE ( 'NONE', *, *, #3516, .F. ) ;
#8713=CARTESIAN_POINT ( 'NONE',  ( -12.84999999999999964, -2.000000000000001776, 2.549999999999997158 ) ) ;
#8714=CARTESIAN_POINT ( 'NONE',  ( 10.50000000000000888, -2.000000000000001776, 5.750000000000005329 ) ) ;
#8730=DIRECTION ( 'NONE',  ( 5.551115123125818447E-17, 6.982962677686276177E-15, 1.000000000000000000 ) ) ;
#8731=AXIS2_PLACEMENT_3D ( 'NONE', #3447, #48, #2021 ) ;
#8740=CARTESIAN_POINT ( 'NONE',  ( -8.954763739086851970, -0.5000000000000004441, 6.678571428571422608 ) ) ;
#8742=AXIS2_PLACEMENT_3D ( 'NONE', #5826, #2275, #9573 ) ;
#8751=EDGE_LOOP ( 'NONE', ( #9681, #8444, #22527, #21835 ) ) ;
#8752=ORIENTED_EDGE ( 'NONE', *, *, #16549, .F. ) ;
#8754=AXIS2_PLACEMENT_3D ( 'NONE', #12836, #18138, #18253 ) ;
#8774=CIRCLE ( 'NONE', #21929, 4.000000000000000000 ) ;
#8777=CARTESIAN_POINT ( 'NONE',  ( -8.113551354209993960, -1.583389928980782457, 7.426820295479581446 ) ) ;
#8801=FACE_OUTER_BOUND ( 'NONE', #20663, .T. ) ;
#8802=FACE_OUTER_BOUND ( 'NONE', #1754, .T. ) ;
#8806=EDGE_CURVE ( 'NONE', #9602, #4343, #21447, .T. ) ;
#8831=CARTESIAN_POINT ( 'NONE',  ( -7.028413389564965641, -13.36994781876315130, 8.946655872546031674 ) ) ;
#8833=CARTESIAN_POINT ( 'NONE',  ( 8.422565759993842605, -1.999999999999981792, 6.396710472006605919 ) ) ;
#8843=VECTOR ( 'NONE', #13881, 1000.000000000000000 ) ;
#8851=FACE_OUTER_BOUND ( 'NONE', #7372, .T. ) ;
#8857=CARTESIAN_POINT ( 'NONE',  ( 7.499999999999979572, -12.77629584335316437, 9.030675447289000957 ) ) ;
#8863=CARTESIAN_POINT ( 'NONE',  ( 12.84999999999997300, -1.499999999999997780, 1.387778780781445676E-14 ) ) ;
#8868=EDGE_LOOP ( 'NONE', ( #11084, #10961, #3607, #21897 ) ) ;
#8876=ORIENTED_EDGE ( 'NONE', *, *, #5784, .F. ) ;
#8882=CARTESIAN_POINT ( 'NONE',  ( -8.137537312224766950, -13.43749107754207017, 7.396067884835361816 ) ) ;
#8904=ORIENTED_EDGE ( 'NONE', *, *, #17112, .F. ) ;
#8907=EDGE_LOOP ( 'NONE', ( #1187, #17066, #15245, #20711 ) ) ;
#8927=VERTEX_POINT ( 'NONE', #16570 ) ;
#8942=DIRECTION ( 'NONE',  ( 5.551115123125818447E-17, -1.577721810442025713E-30, 1.000000000000000000 ) ) ;
#8947=DIRECTION ( 'NONE',  ( 0.000000000000000000, 0.000000000000000000, -1.000000000000000000 ) ) ;
#8955=VERTEX_POINT ( 'NONE', #20125 ) ;
#8961=ORIENTED_EDGE ( 'NONE', *, *, #16881, .T. ) ;
#8969=CARTESIAN_POINT ( 'NONE',  ( -10.49999999999998224, -0.5000000000000038858, 6.250000000000061284 ) ) ;
#8972=DIRECTION ( 'NONE',  ( 0.000000000000000000, 0.000000000000000000, 1.000000000000000000 ) ) ;
#8979=DIRECTION ( 'NONE',  ( 0.000000000000000000, 0.000000000000000000, 1.000000000000000000 ) ) ;
#8983=EDGE_CURVE ( 'NONE', #6938, #23124, #523, .T. ) ;
#8986=CARTESIAN_POINT ( 'NONE',  ( 7.991520206789727965, -0.6043476454135817688, 7.599114430427888145 ) ) ;
#8996=AXIS2_PLACEMENT_3D ( 'NONE', #3833, #19963, #4294 ) ;
#9003=CARTESIAN_POINT ( 'NONE',  ( -8.502135871254331789, -13.49242826152325492, 6.995667647939170841 ) ) ;
#9006=CARTESIAN_POINT ( 'NONE',  ( -10.49999999999996803, -12.50000000000002842, 5.750000000000060396 ) ) ;
#9011=CARTESIAN_POINT ( 'NONE',  ( -7.713464495931991571, -1.828647720521560327, 8.131426806228610360 ) ) ;
#9021=ORIENTED_EDGE ( 'NONE', *, *, #8539, .F. ) ;
#9031=CARTESIAN_POINT ( 'NONE',  ( 7.595478965369733437, -11.97605770252014246, 8.489833260407458226 ) ) ;
#9034=DIRECTION ( 'NONE',  ( 1.000000000000000000, 6.224605580259554159E-31, -2.887593071917436153E-31 ) ) ;
#9040=VERTEX_POINT ( 'NONE', #4817 ) ;
#9052=CARTESIAN_POINT ( 'NONE',  ( -7.126417736726679664, -13.56697759857014596, 8.494066294656329674 ) ) ;
#9069=AXIS2_PLACEMENT_3D ( 'NONE', #14321, #1731, #19741 ) ;
#9073=CARTESIAN_POINT ( 'NONE',  ( 7.835522544085312902, -11.94917567266014480, 6.894286109559232045 ) ) ;
#9077=CARTESIAN_POINT ( 'NONE',  ( 8.223343937052064234, -13.45452499186315265, 7.291631794411112644 ) ) ;
#9086=ADVANCED_FACE ( 'NONE', ( #2947 ), #20049, .T. ) ;
#9095=ORIENTED_EDGE ( 'NONE', *, *, #22846, .F. ) ;
#9099=ORIENTED_EDGE ( 'NONE', *, *, #877, .T. ) ;
#9101=ORIENTED_EDGE ( 'NONE', *, *, #10964, .F. ) ;
#9103=EDGE_CURVE ( 'NONE', #11691, #6938, #18704, .T. ) ;
#9109=AXIS2_PLACEMENT_3D ( 'NONE', #17490, #13744, #10096 ) ;
#9138=DIRECTION ( 'NONE',  ( 0.000000000000000000, 0.000000000000000000, -1.000000000000000000 ) ) ;
#9141=VECTOR ( 'NONE', #11742, 1000.000000000000000 ) ;
#9145=CARTESIAN_POINT ( 'NONE',  ( -7.499999999999992895, -8.000000000000044409, 6.250000000000005329 ) ) ;
#9147=EDGE_CURVE ( 'NONE', #9714, #4863, #16287, .T. ) ;
#9152=CARTESIAN_POINT ( 'NONE',  ( -7.694134585029390294, -13.68800912542550385, 8.172315317061205064 ) ) ;
#9176=CARTESIAN_POINT ( 'NONE',  ( 7.554637128289433790, -13.87985946887537558, 7.453047528892627227 ) ) ;
#9177=CARTESIAN_POINT ( 'NONE',  ( 8.178874953434442929, -13.99214848402183797, 6.644730819939103306 ) ) ;
#9178=CARTESIAN_POINT ( 'NONE',  ( -12.84999999999999964, -14.00000000000003020, 5.750000000000032863 ) ) ;
#9185=ORIENTED_EDGE ( 'NONE', *, *, #20527, .F. ) ;
#9187=EDGE_CURVE ( 'NONE', #20539, #9220, #7064, .T. ) ;
#9196=CARTESIAN_POINT ( 'NONE',  ( 8.954763739086837759, -12.50000000000004619, 6.678571428571492774 ) ) ;
#9200=DIRECTION ( 'NONE',  ( 0.000000000000000000, 0.000000000000000000, 1.000000000000000000 ) ) ;
#9204=DIRECTION ( 'NONE',  ( -0.5150787536377134934, 0.000000000000000000, 0.8571428571428567622 ) ) ;
#9207=DIRECTION ( 'NONE',  ( 0.000000000000000000, -7.888609052210126812E-31, 1.000000000000000000 ) ) ;
#9212=CARTESIAN_POINT ( 'NONE',  ( 8.954763739086837759, -0.4999999999999852895, 6.678571428571446589 ) ) ;
#9220=VERTEX_POINT ( 'NONE', #6819 ) ;
#9248=EDGE_CURVE ( 'NONE', #1201, #8077, #12908, .T. ) ;
#9263=CARTESIAN_POINT ( 'NONE',  ( -7.000000000000020428, -3.018576030000264865, 8.916666666666712260 ) ) ;
#9271=DIRECTION ( 'NONE',  ( 0.000000000000000000, 0.000000000000000000, 1.000000000000000000 ) ) ;
#9279=DIRECTION ( 'NONE',  ( 1.000000000000000000, 4.252453317207022018E-31, -5.551115123125818447E-17 ) ) ;
#9291=CIRCLE ( 'NONE', #12278, 0.4999999999999995559 ) ;
#9302=VERTEX_POINT ( 'NONE', #14568 ) ;
#9303=AXIS2_PLACEMENT_3D ( 'NONE', #9439, #7784, #848 ) ;
#9309=CARTESIAN_POINT ( 'NONE',  ( 7.500000000000007994, -11.57130297832598309, 9.041853041260921486 ) ) ;
#9310=DIRECTION ( 'NONE',  ( -4.019602852144215652E-47, -6.982962677686261977E-15, -1.000000000000000000 ) ) ;
#9329=CARTESIAN_POINT ( 'NONE',  ( 8.115139842999449016, -0.1079360712687435775, 7.423524081915865658 ) ) ;
#9332=VERTEX_POINT ( 'NONE', #7401 ) ;
#9347=CARTESIAN_POINT ( 'NONE',  ( -7.670621117724356175, -2.511599330828965027, 8.215271161873788586 ) ) ;
#9363=ORIENTED_EDGE ( 'NONE', *, *, #6808, .T. ) ;
#9364=ORIENTED_EDGE ( 'NONE', *, *, #10964, .T. ) ;
#9370=VERTEX_POINT ( 'NONE', #3741 ) ;
#9374=EDGE_CURVE ( 'NONE', #21109, #280, #15533, .T. ) ;
#9378=LINE ( 'NONE', #4536, #14701 ) ;
#9392=B_SPLINE_CURVE_WITH_KNOTS ( 'NONE', 3,
 ( #8673, #10667, #15027, #21396, #19495, #22797, #12545, #3391, #13958, #17969, #16065, #5022, #14208, #15830 ),
 .UNSPECIFIED., .F., .F.,
 ( 4, 2, 2, 2, 2, 2, 4 ),
 ( 0.000000000000000000, 0.0008249779604813560832, 0.001237466940722032173, 0.001649955920962708480, 0.002062444901203385871, 0.002474933881444063913, 0.003299911841925418261 ),
 .UNSPECIFIED. ) ;
#9394=LINE ( 'NONE', #21981, #15500 ) ;
#9404=FACE_OUTER_BOUND ( 'NONE', #15630, .T. ) ;
#9411=CARTESIAN_POINT ( 'NONE',  ( 7.694134585029463125, -13.68800912542550741, 8.172315317061212170 ) ) ;
#9416=DIRECTION ( 'NONE',  ( -1.000000000000000000, -1.910522504832140594E-31, 5.551115123125818447E-17 ) ) ;
#9417=ADVANCED_FACE ( 'NONE', ( #15253 ), #10094, .T. ) ;
#9431=DIRECTION ( 'NONE',  ( 1.000000000000000000, 4.252453317207022018E-31, -5.551115123125818447E-17 ) ) ;
#9436=CARTESIAN_POINT ( 'NONE',  ( -12.85000000000002807, -1.999999999999998224, 6.249999999999950262 ) ) ;
#9439=CARTESIAN_POINT ( 'NONE',  ( 6.999999999999992006, -8.000000000000051514, 6.249999999999977796 ) ) ;
#9441=CARTESIAN_POINT ( 'NONE',  ( 7.876571740167059410, -0.1939399797844648943, 7.785394814390983242 ) ) ;
#9475=ORIENTED_EDGE ( 'NONE', *, *, #16518, .T. ) ;
#9481=ORIENTED_EDGE ( 'NONE', *, *, #915, .F. ) ;
#9487=CARTESIAN_POINT ( 'NONE',  ( 8.697224362267997222, -1.499999999999984013, 6.250000000000005329 ) ) ;
#9488=CARTESIAN_POINT ( 'NONE',  ( -7.029812747553743080, -13.37717092480936643, 8.933015330925142550 ) ) ;
#9491=CARTESIAN_POINT ( 'NONE',  ( 8.715898959466906959, -1.502431622389267751, 6.833978265954022469 ) ) ;
#9508=CIRCLE ( 'NONE', #17798, 2.999999999999995559 ) ;
#9513=ADVANCED_FACE ( 'NONE', ( #13387 ), #11960, .F. ) ;
#9541=CARTESIAN_POINT ( 'NONE',  ( 8.697224362267972353, -12.00000000000004796, 6.250000000000059508 ) ) ;
#9543=EDGE_CURVE ( 'NONE', #20452, #9827, #9859, .T. ) ;
#9556=CARTESIAN_POINT ( 'NONE',  ( 6.999999999999992006, -5.999999999999981348, 10.74999999999998224 ) ) ;
#9558=B_SPLINE_CURVE_WITH_KNOTS ( 'NONE', 3,
 ( #2812, #2683, #6891, #23008, #3372, #6111, #10414, #9870, #21254, #15696, #21128, #20578, #22346, #12281 ),
 .UNSPECIFIED., .F., .F.,
 ( 4, 2, 2, 2, 2, 2, 4 ),
 ( 0.000000000000000000, 0.0008155857435326423210, 0.001223378615298963265, 0.001631171487065284642, 0.002038964358831601032, 0.002446757230597917422, 0.003262342974130546733 ),
 .UNSPECIFIED. ) ;
#9568=ORIENTED_EDGE ( 'NONE', *, *, #8436, .F. ) ;
#9571=VERTEX_POINT ( 'NONE', #22919 ) ;
#9572=EDGE_CURVE ( 'NONE', #635, #10026, #9392, .T. ) ;
#9573=DIRECTION ( 'NONE',  ( 1.665334536937736980E-15, 0.000000000000000000, 1.000000000000000000 ) ) ;
#9580=EDGE_CURVE ( 'NONE', #10962, #3180, #12064, .T. ) ;
#9583=AXIS2_PLACEMENT_3D ( 'NONE', #17428, #23099, #14021 ) ;
#9602=VERTEX_POINT ( 'NONE', #17851 ) ;
#9605=CARTESIAN_POINT ( 'NONE',  ( -12.85000000000005649, -12.50000000000011191, -6.249999999999921840 ) ) ;
#9607=CARTESIAN_POINT ( 'NONE',  ( -12.84999999999999964, -2.000000000000001776, 0.000000000000000000 ) ) ;
#9609=CARTESIAN_POINT ( 'NONE',  ( -8.129778652391308924, -12.42126101213639444, 7.405931224841348026 ) ) ;
#9617=DIRECTION ( 'NONE',  ( -1.000000000000000000, -6.224605580259554159E-31, 2.887593071917436153E-31 ) ) ;
#9627=DIRECTION ( 'NONE',  ( 5.551115123125761132E-17, -1.577721810442025713E-30, 1.000000000000000000 ) ) ;
#9632=CARTESIAN_POINT ( 'NONE',  ( 7.126417736726686769, -13.56697759857014418, 8.494066294656340332 ) ) ;
#9637=( LENGTH_UNIT ( ) NAMED_UNIT ( * ) SI_UNIT ( .MILLI., .METRE. ) );
#9654=DIRECTION ( 'NONE',  ( 3.862887998903635106E-15, -0.5454545454545466354, 0.8381404052084434619 ) ) ;
#9664=CIRCLE ( 'NONE', #6283, 0.4999999999999995559 ) ;
#9668=DIRECTION ( 'NONE',  ( 9.121204216617949000E-31, 1.000000000000000000, -6.982962677686261977E-15 ) ) ;
#9681=ORIENTED_EDGE ( 'NONE', *, *, #23225, .F. ) ;
#9689=AXIS2_PLACEMENT_3D ( 'NONE', #15495, #8220, #11859 ) ;
#9692=CARTESIAN_POINT ( 'NONE',  ( -7.499999999999989342, -2.428697021683995594, 9.041853041250330847 ) ) ;
#9704=ADVANCED_FACE ( 'NONE', ( #20309 ), #11244, .F. ) ;
#9705=DIRECTION ( 'NONE',  ( 6.656013887802287108E-31, 1.000000000000000000, -3.469446951953609061E-15 ) ) ;
#9710=VERTEX_POINT ( 'NONE', #16520 ) ;
#9714=VERTEX_POINT ( 'NONE', #11006 ) ;
#9717=VERTEX_POINT ( 'NONE', #5962 ) ;
#9721=VERTEX_POINT ( 'NONE', #431 ) ;
#9727=FACE_OUTER_BOUND ( 'NONE', #2036, .T. ) ;
#9729=CARTESIAN_POINT ( 'NONE',  ( -7.282868595548766422, -13.73825694947798581, 8.010178330700920668 ) ) ;
#9730=AXIS2_PLACEMENT_3D ( 'NONE', #19860, #7170, #16318 ) ;
#9738=B_SPLINE_CURVE_WITH_KNOTS ( 'NONE', 3,
 ( #3097, #21453, #12481, #5322, #5210, #1337, #19325, #10725, #12369, #15660, #19552, #1219, #22860, #6737 ),
 .UNSPECIFIED., .F., .F.,
 ( 4, 2, 2, 2, 2, 2, 4 ),
 ( 2.826448204503814216E-21, 0.001011182963765816078, 0.001516774445648722165, 0.002022365927531628253, 0.002527957409414534340, 0.003033548891297440427, 0.004044731855063248699 ),
 .UNSPECIFIED. ) ;
#9756=DIRECTION ( 'NONE',  ( 0.000000000000000000, 6.938893903907245733E-15, 1.000000000000000000 ) ) ;
#9766=EDGE_LOOP ( 'NONE', ( #10286, #9475, #20916, #3294 ) ) ;
#9767=EDGE_LOOP ( 'NONE', ( #5198, #20893, #8290, #15453 ) ) ;
#9773=DIRECTION ( 'NONE',  ( 1.927470528863118556E-16, 1.000000000000000000, -7.131640956793539050E-15 ) ) ;
#9780=CARTESIAN_POINT ( 'NONE',  ( 10.50000000000000888, -1.500000000000001332, 9.250000000000008882 ) ) ;
#9789=UNCERTAINTY_MEASURE_WITH_UNIT (LENGTH_MEASURE( 1.000000000000000082E-05 ), #15597, 'distance_accuracy_value', 'NONE');
#9801=DIRECTION ( 'NONE',  ( -9.121204216617949000E-31, -1.000000000000000000, 6.982962677686261977E-15 ) ) ;
#9808=CARTESIAN_POINT ( 'NONE',  ( 7.778057173929710189, -1.762098510204312518, 7.981635986975429198 ) ) ;
#9827=VERTEX_POINT ( 'NONE', #2532 ) ;
#9831=EDGE_CURVE ( 'NONE', #9302, #2116, #10222, .T. ) ;
#9838=DIRECTION ( 'NONE',  ( -1.000000000000000000, 2.168404344971005170E-16, -1.203141491611682442E-30 ) ) ;
#9839=CARTESIAN_POINT ( 'NONE',  ( -8.954763739086832430, -12.00000000000004263, 6.678571428571464352 ) ) ;
#9841=FACE_BOUND ( 'NONE', #5103, .T. ) ;
#9859=LINE ( 'NONE', #17016, #1958 ) ;
#9870=CARTESIAN_POINT ( 'NONE',  ( -7.909386411296974728, -0.6370970679665923786, 7.731447622712464884 ) ) ;
#9885=VECTOR ( 'NONE', #17659, 1000.000000000000000 ) ;
#9895=CARTESIAN_POINT ( 'NONE',  ( -7.499999999999992895, -5.999999999999987566, 6.249999999999992006 ) ) ;
#9897=FACE_OUTER_BOUND ( 'NONE', #17244, .T. ) ;
#9913=ORIENTED_EDGE ( 'NONE', *, *, #4970, .T. ) ;
#9915=CIRCLE ( 'NONE', #5789, 5.749999999999992006 ) ;
#9922=CYLINDRICAL_SURFACE ( 'NONE', #11048, 0.4999999999999987232 ) ;
#9927=CARTESIAN_POINT ( 'NONE',  ( -7.854293383767849690, -2.312270958411835498, 7.820081954006687042 ) ) ;
#9948=EDGE_CURVE ( 'NONE', #18911, #8641, #16995, .T. ) ;
#9961=CARTESIAN_POINT ( 'NONE',  ( 12.84999999999997300, -12.00000000000002842, 5.750000000000018652 ) ) ;
#9963=CARTESIAN_POINT ( 'NONE',  ( -8.721922330811601398, -13.98762810781391686, 6.818491697976370780 ) ) ;
#9964=EDGE_CURVE ( 'NONE', #2238, #15768, #4219, .T. ) ;
#9975=VERTEX_POINT ( 'NONE', #18887 ) ;
#9979=DIRECTION ( 'NONE',  ( -1.454462294001240516E-30, -1.000000000000000000, -0.000000000000000000 ) ) ;
#9985=AXIS2_PLACEMENT_3D ( 'NONE', #19872, #3531, #14112 ) ;
#9992=DIRECTION ( 'NONE',  ( 3.469446951953611428E-15, -1.000000000000000000, 3.469446951953610245E-15 ) ) ;
#10003=VECTOR ( 'NONE', #9627, 1000.000000000000000 ) ;
#10006=CIRCLE ( 'NONE', #23170, 6.249999999999992006 ) ;
#10015=FACE_OUTER_BOUND ( 'NONE', #4600, .T. ) ;
#10025=CIRCLE ( 'NONE', #22413, 0.4999999999999998335 ) ;
#10026=VERTEX_POINT ( 'NONE', #17825 ) ;
#10035=DIRECTION ( 'NONE',  ( 1.000000000000000000, 6.224605580259554159E-31, -2.887593071917436153E-31 ) ) ;
#10037=CARTESIAN_POINT ( 'NONE',  ( -8.697224362267958142, -1.999999999999988010, 6.249999999999968914 ) ) ;
#10041=CARTESIAN_POINT ( 'NONE',  ( 7.802869476033482243, -2.356467536663165330, 7.917139222843119661 ) ) ;
#10069=FACE_OUTER_BOUND ( 'NONE', #23123, .T. ) ;
#10089=ORIENTED_EDGE ( 'NONE', *, *, #15414, .T. ) ;
#10094=CYLINDRICAL_SURFACE ( 'NONE', #8369, 0.4999999999999995559 ) ;
#10096=DIRECTION ( 'NONE',  ( 0.000000000000000000, 0.000000000000000000, 1.000000000000000000 ) ) ;
#10102=CARTESIAN_POINT ( 'NONE',  ( -7.613388670473234754, -0.8883455870200124282, 8.423574099071704069 ) ) ;
#10105=EDGE_CURVE ( 'NONE', #21109, #11093, #12115, .T. ) ;
#10114=AXIS2_PLACEMENT_3D ( 'NONE', #21259, #15934, #7143 ) ;
#10122=DIRECTION ( 'NONE',  ( -1.000000000000000000, -2.312964634635752325E-16, 1.880120159248731926E-30 ) ) ;
#10123=DIRECTION ( 'NONE',  ( 9.121204216617949000E-31, 1.000000000000000000, -6.982962677686261977E-15 ) ) ;
#10127=ADVANCED_FACE ( 'NONE', ( #19580 ), #21004, .T. ) ;
#10128=CYLINDRICAL_SURFACE ( 'NONE', #1175, 0.4999999999999995559 ) ;
#10152=CARTESIAN_POINT ( 'NONE',  ( -7.835522544085302243, -2.050824327339882736, 6.894286109559143227 ) ) ;
#10155=CARTESIAN_POINT ( 'NONE',  ( 7.568091547083615644, -2.695633093450964246, 8.516664522245834590 ) ) ;
#10157=CARTESIAN_POINT ( 'NONE',  ( -12.84999999999999964, -2.000000000000001776, 5.750000000000005329 ) ) ;
#10193=EDGE_LOOP ( 'NONE', ( #2289, #10312, #14505, #21889 ) ) ;
#10203=CARTESIAN_POINT ( 'NONE',  ( -8.429621201837308675, 1.266960025302491611E-14, 6.425428529985098614 ) ) ;
#10205=DIRECTION ( 'NONE',  ( 1.000000000000000000, -2.168404344971005170E-16, 1.203141491611682442E-30 ) ) ;
#10222=CIRCLE ( 'NONE', #13237, 2.549999999999997158 ) ;
#10227=EDGE_LOOP ( 'NONE', ( #2585, #21300, #18022, #17456 ) ) ;
#10243=VECTOR ( 'NONE', #4087, 1000.000000000000000 ) ;
#10254=ORIENTED_EDGE ( 'NONE', *, *, #12245, .F. ) ;
#10257=PLANE ( 'NONE',  #9583 ) ;
#10258=DIRECTION ( 'NONE',  ( -5.546678239835239257E-32, -1.000000000000000000, 6.938893903907215756E-15 ) ) ;
#10281=CIRCLE ( 'NONE', #7665, 6.249999999999992006 ) ;
#10286=ORIENTED_EDGE ( 'NONE', *, *, #16090, .T. ) ;
#10288=DIRECTION ( 'NONE',  ( 0.000000000000000000, -6.938893903907237055E-15, -1.000000000000000000 ) ) ;
#10296=DIRECTION ( 'NONE',  ( -1.232595164407830946E-32, 1.000000000000000000, -6.938893903907214967E-15 ) ) ;
#10304=ORIENTED_EDGE ( 'NONE', *, *, #19029, .T. ) ;
#10312=ORIENTED_EDGE ( 'NONE', *, *, #16981, .T. ) ;
#10321=DIRECTION ( 'NONE',  ( -9.121204216617949000E-31, -1.000000000000000000, 6.982962677686261977E-15 ) ) ;
#10324=CARTESIAN_POINT ( 'NONE',  ( -6.999999995197900837, -0.7826352830280864925, 9.233045673661063546 ) ) ;
#10330=CARTESIAN_POINT ( 'NONE',  ( 7.500000000000007105, -5.999999999999981348, 11.74999999999995559 ) ) ;
#10338=ORIENTED_EDGE ( 'NONE', *, *, #4921, .F. ) ;
#10340=DIRECTION ( 'NONE',  ( 1.454462294001240516E-30, 1.000000000000000000, 0.000000000000000000 ) ) ;
#10348=DIRECTION ( 'NONE',  ( 1.454462294001240516E-30, 1.000000000000000000, 0.000000000000000000 ) ) ;
#10359=VERTEX_POINT ( 'NONE', #20396 ) ;
#10362=EDGE_LOOP ( 'NONE', ( #6788, #5107, #1778, #21784 ) ) ;
#10367=VERTEX_POINT ( 'NONE', #13770 ) ;
#10386=DIRECTION ( 'NONE',  ( 0.000000000000000000, -6.938893903907237844E-15, -1.000000000000000000 ) ) ;
#10392=ORIENTED_EDGE ( 'NONE', *, *, #22201, .T. ) ;
#10410=CARTESIAN_POINT ( 'NONE',  ( 12.84999999999998721, -13.50000000000003020, 6.250000000000033751 ) ) ;
#10414=CARTESIAN_POINT ( 'NONE',  ( -7.786490775660069197, -0.7065074219475123707, 7.963863235126036777 ) ) ;
#10416=ADVANCED_FACE ( 'NONE', ( #10579 ), #23072, .T. ) ;
#10445=CARTESIAN_POINT ( 'NONE',  ( -7.500000000000016875, -1.217419751679961415, 9.022398393216642276 ) ) ;
#10455=DIRECTION ( 'NONE',  ( 0.000000000000000000, 0.000000000000000000, 1.000000000000000000 ) ) ;
#10463=VERTEX_POINT ( 'NONE', #21302 ) ;
#10470=VERTEX_POINT ( 'NONE', #10471 ) ;
#10471=CARTESIAN_POINT ( 'NONE',  ( 10.50000000000000888, -12.00000000000002842, 5.750000000000032863 ) ) ;
#10473=CARTESIAN_POINT ( 'NONE',  ( 10.50000000000000888, -12.50000000000002842, 6.250000000000061284 ) ) ;
#10487=ORIENTED_EDGE ( 'NONE', *, *, #12959, .T. ) ;
#10495=DIRECTION ( 'NONE',  ( 3.469446951953619316E-15, -6.938893903907238633E-15, -1.000000000000000000 ) ) ;
#10512=ORIENTED_EDGE ( 'NONE', *, *, #8442, .F. ) ;
#10516=ORIENTED_EDGE ( 'NONE', *, *, #14197, .T. ) ;
#10520=ORIENTED_EDGE ( 'NONE', *, *, #7676, .T. ) ;
#10526=DIRECTION ( 'NONE',  ( 1.000000000000000000, 2.168404344971017743E-16, -1.780660105995169760E-30 ) ) ;
#10530=CARTESIAN_POINT ( 'NONE',  ( -12.84999999999999964, -2.000000000000001776, 0.000000000000000000 ) ) ;
#10543=EDGE_LOOP ( 'NONE', ( #13326, #4785, #7349, #13483 ) ) ;
#10556=FACE_OUTER_BOUND ( 'NONE', #21983, .T. ) ;
#10557=FACE_OUTER_BOUND ( 'NONE', #12540, .T. ) ;
#10564=CARTESIAN_POINT ( 'NONE',  ( 12.84999999999997300, -2.000000000000001776, -6.249999999999992006 ) ) ;
#10568=ORIENTED_EDGE ( 'NONE', *, *, #22338, .T. ) ;
#10579=FACE_OUTER_BOUND ( 'NONE', #4372, .T. ) ;
#10583=DIRECTION ( 'NONE',  ( 0.000000000000000000, 0.000000000000000000, 1.000000000000000000 ) ) ;
#10606=CARTESIAN_POINT ( 'NONE',  ( 7.607945571813336194, -13.10245601331112653, 8.443122311927350410 ) ) ;
#10617=CARTESIAN_POINT ( 'NONE',  ( 7.491585531133562625, -2.143791077336254514, 7.320610673787141920 ) ) ;
#10627=ORIENTED_EDGE ( 'NONE', *, *, #8373, .T. ) ;
#10628=AXIS2_PLACEMENT_3D ( 'NONE', #14372, #14494, #19431 ) ;
#10642=DIRECTION ( 'NONE',  ( 0.000000000000000000, 6.938893903907237055E-15, 1.000000000000000000 ) ) ;
#10650=CARTESIAN_POINT ( 'NONE',  ( -8.200527591913209235, -1.560621988374211178, 7.318116290495742859 ) ) ;
#10660=EDGE_LOOP ( 'NONE', ( #15915, #22651, #15745, #313 ) ) ;
#10661=ADVANCED_FACE ( 'NONE', ( #11497 ), #3521, .T. ) ;
#10667=CARTESIAN_POINT ( 'NONE',  ( 8.718376657154808029, -0.4999999999999831246, 6.820622386031985229 ) ) ;
#10669=DIRECTION ( 'NONE',  ( 0.000000000000000000, -3.469446951953622866E-15, -1.000000000000000000 ) ) ;
#10671=EDGE_CURVE ( 'NONE', #11093, #5891, #16333, .T. ) ;
#10675=CARTESIAN_POINT ( 'NONE',  ( 8.954763739086866181, -12.50000000000002132, 6.678571428571491886 ) ) ;
#10704=FACE_OUTER_BOUND ( 'NONE', #13474, .T. ) ;
#10709=CARTESIAN_POINT ( 'NONE',  ( 7.500000000000007105, -11.35410196624971491, 9.250000000000021316 ) ) ;
#10717=ORIENTED_EDGE ( 'NONE', *, *, #20136, .F. ) ;
#10721=CARTESIAN_POINT ( 'NONE',  ( 7.670621117724267357, -11.48840066917087022, 8.215271161873694439 ) ) ;
#10725=CARTESIAN_POINT ( 'NONE',  ( -7.332081355611433260, -0.2267865287842164845, 7.890992604157045065 ) ) ;
#10726=CARTESIAN_POINT ( 'NONE',  ( 8.137537312224765174, -13.43749107754207017, 7.396067884835384021 ) ) ;
#10743=ORIENTED_EDGE ( 'NONE', *, *, #17473, .F. ) ;
#10745=ORIENTED_EDGE ( 'NONE', *, *, #11252, .F. ) ;
#10753=CARTESIAN_POINT ( 'NONE',  ( -8.223343937052071340, -13.45452499186315443, 7.291631794411082446 ) ) ;
#10775=AXIS2_PLACEMENT_3D ( 'NONE', #8863, #8512, #49 ) ;
#10788=DIRECTION ( 'NONE',  ( -9.121204216617949000E-31, -1.000000000000000000, 6.982962677686261977E-15 ) ) ;
#10795=DIRECTION ( 'NONE',  ( 6.656013887802287108E-31, 1.000000000000000000, -3.469446951953609061E-15 ) ) ;
#10809=AXIS2_PLACEMENT_3D ( 'NONE', #12613, #1690, #16135 ) ;
#10818=CARTESIAN_POINT ( 'NONE',  ( 8.518530740349840258, -2.043531002858649082, 6.984205661427222545 ) ) ;
#10825=EDGE_CURVE ( 'NONE', #9571, #17483, #17369, .T. ) ;
#10827=EDGE_CURVE ( 'NONE', #19001, #19925, #5501, .T. ) ;
#10832=EDGE_LOOP ( 'NONE', ( #15311, #10304, #15338, #22736, #20620, #4727, #4953, #9364 ) ) ;
#10835=ADVANCED_FACE ( 'NONE', ( #12660 ), #1961, .T. ) ;
#10838=CARTESIAN_POINT ( 'NONE',  ( 8.216162181246577489, -12.44282262938666328, 7.299847320220921532 ) ) ;
#10852=DIRECTION ( 'NONE',  ( 1.454462294001240516E-30, 1.000000000000000000, 0.000000000000000000 ) ) ;
#10854=CARTESIAN_POINT ( 'NONE',  ( 7.951003271401690498, -0.1617022081438048986, 7.659883344695789020 ) ) ;
#10857=VERTEX_POINT ( 'NONE', #15730 ) ;
#10859=AXIS2_PLACEMENT_3D ( 'NONE', #14074, #21263, #12533 ) ;
#10870=CARTESIAN_POINT ( 'NONE',  ( 12.84999999999997300, -13.50000000000007105, 5.551115123125782702E-14 ) ) ;
#10898=CARTESIAN_POINT ( 'NONE',  ( -8.697224362268011433, -14.00000000000004441, 6.250000000000033751 ) ) ;
#10903=CARTESIAN_POINT ( 'NONE',  ( -7.499999999999992895, -5.999999999999987566, 6.249999999999992006 ) ) ;
#10918=CARTESIAN_POINT ( 'NONE',  ( 8.233775472210654200, -13.45629277298760584, 7.279685395985904250 ) ) ;
#10919=CARTESIAN_POINT ( 'NONE',  ( 8.954763739086866181, -1.999999999999987343, 6.678571428571431490 ) ) ;
#10920=CIRCLE ( 'NONE', #15066, 0.4999999999999995559 ) ;
#10928=EDGE_CURVE ( 'NONE', #19419, #7917, #4205, .T. ) ;
#10937=CIRCLE ( 'NONE', #15458, 4.000000000000000000 ) ;
#10941=CARTESIAN_POINT ( 'NONE',  ( 8.498922697886598598, -12.49080420435820926, 6.997949321565184455 ) ) ;
#10942=CARTESIAN_POINT ( 'NONE',  ( -7.162073728446670451, -11.63471678239051954, 7.945145523438286617 ) ) ;
#10961=ORIENTED_EDGE ( 'NONE', *, *, #16981, .F. ) ;
#10962=VERTEX_POINT ( 'NONE', #14212 ) ;
#10964=EDGE_CURVE ( 'NONE', #15768, #9602, #15106, .T. ) ;
#10971=CARTESIAN_POINT ( 'NONE',  ( 7.000000000000020428, -13.02884243125069652, 9.522727272727321335 ) ) ;
#10972=EDGE_LOOP ( 'NONE', ( #16545, #22232, #16000, #20738, #6359, #21497 ) ) ;
#10974=CARTESIAN_POINT ( 'NONE',  ( -12.84999999999999964, -0.5000000000000004441, -5.749999999999963585 ) ) ;
#10981=VECTOR ( 'NONE', #12304, 1000.000000000000000 ) ;
#10988=VECTOR ( 'NONE', #501, 1000.000000000000000 ) ;
#10999=VECTOR ( 'NONE', #17830, 1000.000000000000000 ) ;
#11006=CARTESIAN_POINT ( 'NONE',  ( 8.954763739086866181, -12.50000000000002132, 6.678571428571491886 ) ) ;
#11018=CARTESIAN_POINT ( 'NONE',  ( -7.499999999999994671, -13.02884243125068586, 9.522727272727351533 ) ) ;
#11023=LINE ( 'NONE', #11359, #19028 ) ;
#11037=CARTESIAN_POINT ( 'NONE',  ( 7.761744141695591459, -11.93564195219169299, 6.973942750959585268 ) ) ;
#11038=PLANE ( 'NONE',  #19603 ) ;
#11045=CARTESIAN_POINT ( 'NONE',  ( 7.525553787417719853, -12.92907334721305368, 8.786654903594133259 ) ) ;
#11048=AXIS2_PLACEMENT_3D ( 'NONE', #16950, #1215, #18977 ) ;
#11052=AXIS2_PLACEMENT_3D ( 'NONE', #14171, #14054, #19347 ) ;
#11055=PRODUCT_CONTEXT ( 'NONE', #12687, 'mechanical' ) ;
#11073=PLANE ( 'NONE',  #2364 ) ;
#11077=CARTESIAN_POINT ( 'NONE',  ( 8.438463404362677167, -2.001835333048895826, 6.398712851742186736 ) ) ;
#11084=ORIENTED_EDGE ( 'NONE', *, *, #12794, .T. ) ;
#11093=VERTEX_POINT ( 'NONE', #9605 ) ;
#11098=CARTESIAN_POINT ( 'NONE',  ( -6.999999999999992006, -3.018576030000268418, 8.916666666666687391 ) ) ;
#11101=CARTESIAN_POINT ( 'NONE',  ( 7.000000000000006217, -1.390227771353540920, 9.250000000000021316 ) ) ;
#11108=DIRECTION ( 'NONE',  ( 0.000000000000000000, 0.7453559924999302311, 0.6666666666666662966 ) ) ;
#11123=DIRECTION ( 'NONE',  ( -1.000000000000000000, -4.252453317207022018E-31, 5.551115123125818447E-17 ) ) ;
#11130=CARTESIAN_POINT ( 'NONE',  ( -6.999999999999992006, -5.999999999999987566, 6.250000000000005329 ) ) ;
#11131=CARTESIAN_POINT ( 'NONE',  ( 7.764145988665070774, -12.22513543353773713, 8.011880279048892106 ) ) ;
#11138=CARTESIAN_POINT ( 'NONE',  ( 12.84999999999997300, -12.00000000000006928, 4.163336342344337027E-14 ) ) ;
#11154=LINE ( 'NONE', #22099, #18280 ) ;
#11166=CARTESIAN_POINT ( 'NONE',  ( 7.796097383573778572, -13.30002726899557253, 7.943830786858248061 ) ) ;
#11170=CARTESIAN_POINT ( 'NONE',  ( 10.50000000000000888, -12.50000000000002842, 6.250000000000061284 ) ) ;
#11178=AXIS2_PLACEMENT_3D ( 'NONE', #9556, #4482, #11537 ) ;
#11182=CARTESIAN_POINT ( 'NONE',  ( 8.160037397871471754, -0.008793114504475355031, 6.662331851011971118 ) ) ;
#11199=DIRECTION ( 'NONE',  ( 1.000000000000000000, -2.168404344971005170E-16, 1.203141491611682442E-30 ) ) ;
#11201=CARTESIAN_POINT ( 'NONE',  ( 7.176407415342007212, -0.3641807091870383761, 8.314790908397654334 ) ) ;
#11209=ORIENTED_EDGE ( 'NONE', *, *, #7371, .T. ) ;
#11210=ORIENTED_EDGE ( 'NONE', *, *, #597, .T. ) ;
#11215=ORIENTED_EDGE ( 'NONE', *, *, #19209, .F. ) ;
#11216=ORIENTED_EDGE ( 'NONE', *, *, #19285, .F. ) ;
#11241=EDGE_CURVE ( 'NONE', #20509, #1546, #21533, .T. ) ;
#11244=CYLINDRICAL_SURFACE ( 'NONE', #23023, 3.999999999999994671 ) ;
#11250=CARTESIAN_POINT ( 'NONE',  ( -7.725871784772736284, -12.18565941508500394, 8.100883686805090633 ) ) ;
#11252=EDGE_CURVE ( 'NONE', #16622, #22329, #5247, .T. ) ;
#11271=LINE ( 'NONE', #13388, #19226 ) ;
#11283=CIRCLE ( 'NONE', #3759, 2.999999999999995559 ) ;
#11294=CIRCLE ( 'NONE', #3050, 4.500000000000000888 ) ;
#11303=CARTESIAN_POINT ( 'NONE',  ( 10.50000000000000888, 0.000000000000000000, 9.249999999999980460 ) ) ;
#11313=ADVANCED_FACE ( 'NONE', ( #23132 ), #15873, .T. ) ;
#11323=CARTESIAN_POINT ( 'NONE',  ( -7.120027569165166881, -2.450222941140165922, 8.099087005775098547 ) ) ;
#11334=VECTOR ( 'NONE', #8163, 1000.000000000000000 ) ;
#11335=CARTESIAN_POINT ( 'NONE',  ( 12.84999999999997300, -14.00000000000008882, -2.549999999999945199 ) ) ;
#11345=DIRECTION ( 'NONE',  ( 0.000000000000000000, 3.469446951953618922E-15, 1.000000000000000000 ) ) ;
#11351=CARTESIAN_POINT ( 'NONE',  ( 12.84999999999997300, -1.500000000000001332, 5.750000000000005329 ) ) ;
#11353=CARTESIAN_POINT ( 'NONE',  ( -7.551224464536113068, -11.87866898603341070, 7.234820221745398960 ) ) ;
#11356=AXIS2_PLACEMENT_3D ( 'NONE', #12633, #17827, #23251 ) ;
#11357=CARTESIAN_POINT ( 'NONE',  ( 8.113551354210041922, -1.583389928980787120, 7.426820295479616973 ) ) ;
#11359=CARTESIAN_POINT ( 'NONE',  ( -10.49999999999995381, -1.499999999999997780, 6.250000000000019540 ) ) ;
#11366=ORIENTED_EDGE ( 'NONE', *, *, #50, .F. ) ;
#11367=ORIENTED_EDGE ( 'NONE', *, *, #16881, .F. ) ;
#11368=CARTESIAN_POINT ( 'NONE',  ( -12.85000000000002807, -1.999999999999998224, 6.249999999999950262 ) ) ;
#11388=CARTESIAN_POINT ( 'NONE',  ( 7.499999999999984013, -13.02884243125068764, 9.522727272727365744 ) ) ;
#11399=AXIS2_PLACEMENT_3D ( 'NONE', #11490, #15488, #2559 ) ;
#11401=ORIENTED_EDGE ( 'NONE', *, *, #12335, .F. ) ;
#11418=DIRECTION ( 'NONE',  ( 1.454462294001240516E-30, 1.000000000000000000, 0.000000000000000000 ) ) ;
#11419=EDGE_CURVE ( 'NONE', #20589, #20148, #21824, .T. ) ;
#11424=DIRECTION ( 'NONE',  ( -1.000000000000000000, -4.252453317207022018E-31, 5.551115123125818447E-17 ) ) ;
#11425=CARTESIAN_POINT ( 'NONE',  ( -12.84999999999999964, -12.00000000000011191, -5.749999999999963585 ) ) ;
#11448=CARTESIAN_POINT ( 'NONE',  ( 7.521298409251896189, -2.242072331701569166, 8.817899680514919680 ) ) ;
#11470=( BOUNDED_SURFACE ( )  B_SPLINE_SURFACE ( 3, 2, ( 
 ( #20208, #11018, #13143 ),
 ( #7497, #4075, #12785 ),
 ( #18430, #2307, #9488 ),
 ( #16418, #21631, #5506 ),
 ( #16651, #563, #20318 ),
 ( #4181, #9152, #9729 ),
 ( #13371, #15120, #20674 ),
 ( #22547, #2660, #2542 ),
 ( #20794, #2781, #6432 ),
 ( #15231, #11594, #1143 ),
 ( #13251, #1023, #794 ),
 ( #19122, #4661, #4298 ),
 ( #16883, #9963, #4538 ),
 ( #15009, #18657, #6201 ) ),
 .UNSPECIFIED., .F., .F., .F. ) 
 B_SPLINE_SURFACE_WITH_KNOTS ( ( 4, 2, 2, 2, 2, 2, 4 ),
 ( 3, 3 ),
 ( 0.000000000000000000, 0.0009385527998839224935, 0.001407829199825883686, 0.001877105599767844987, 0.002346381999709806071, 0.002815658399651767372, 0.003754211199535689974 ),
 ( 0.000000000000000000, 1.000000000000000000 ),
 .UNSPECIFIED. ) 
 GEOMETRIC_REPRESENTATION_ITEM ( )  RATIONAL_B_SPLINE_SURFACE ( (
 ( 1.000000000000000000, 0.7071067811865459074, 1.000000000000000000),
 ( 1.000000000000000000, 0.7217349950158724603, 1.000000000000000000),
 ( 1.000000000000000000, 0.7325631490737404272, 1.000000000000000000),
 ( 1.000000000000000000, 0.7426392126583049036, 1.000000000000000000),
 ( 1.000000000000000000, 0.7449451721693781669, 1.000000000000000000),
 ( 1.000000000000000000, 0.7474053618998787174, 1.000000000000000000),
 ( 1.000000000000000000, 0.7475947887410587800, 1.000000000000000000),
 ( 1.000000000000000000, 0.7461109904165237339, 1.000000000000000000),
 ( 1.000000000000000000, 0.7444113185331598936, 1.000000000000000000),
 ( 1.000000000000000000, 0.7395217850811542926, 1.000000000000000000),
 ( 1.000000000000000000, 0.7363545993504476694, 1.000000000000000000),
 ( 1.000000000000000000, 0.7253814056384388920, 1.000000000000000000),
 ( 1.000000000000000000, 0.7159765610437544003, 1.000000000000000000),
 ( 1.000000000000000000, 0.7071067811865461294, 1.000000000000000000) ) ) 
 REPRESENTATION_ITEM ( '' )  SURFACE ( )  );
#11477=DIRECTION ( 'NONE',  ( 1.927470528863118556E-16, 1.000000000000000000, 0.000000000000000000 ) ) ;
#11486=ORIENTED_EDGE ( 'NONE', *, *, #303, .T. ) ;
#11489=DIRECTION ( 'NONE',  ( 5.551115123125818447E-17, -1.577721810442025713E-30, 1.000000000000000000 ) ) ;
#11490=CARTESIAN_POINT ( 'NONE',  ( 7.000000000000006217, -5.999999999999981348, 6.250000000000005329 ) ) ;
#11491=ORIENTED_EDGE ( 'NONE', *, *, #6824, .T. ) ;
#11497=FACE_OUTER_BOUND ( 'NONE', #7226, .T. ) ;
#11498=DIRECTION ( 'NONE',  ( 0.000000000000000000, 6.802837160693368935E-15, 1.000000000000000000 ) ) ;
#11500=DIRECTION ( 'NONE',  ( 0.000000000000000000, 0.000000000000000000, 1.000000000000000000 ) ) ;
#11509=ORIENTED_EDGE ( 'NONE', *, *, #15166, .F. ) ;
#11518=EDGE_LOOP ( 'NONE', ( #20391, #952, #3690, #7316, #11662, #20680, #14741, #975 ) ) ;
#11520=AXIS2_PLACEMENT_3D ( 'NONE', #7114, #5456, #3570 ) ;
#11523=ORIENTED_EDGE ( 'NONE', *, *, #4401, .F. ) ;
#11536=PLANE ( 'NONE',  #15562 ) ;
#11537=DIRECTION ( 'NONE',  ( 0.000000000000000000, 0.000000000000000000, 1.000000000000000000 ) ) ;
#11544=ORIENTED_EDGE ( 'NONE', *, *, #9964, .F. ) ;
#11545=EDGE_CURVE ( 'NONE', #13819, #6724, #9508, .T. ) ;
#11549=EDGE_CURVE ( 'NONE', #8927, #13556, #7631, .T. ) ;
#11561=CIRCLE ( 'NONE', #21343, 2.549999999999997158 ) ;
#11563=CARTESIAN_POINT ( 'NONE',  ( -6.999999991915156095, -2.825498329575475420, 8.700799235122101294 ) ) ;
#11566=CARTESIAN_POINT ( 'NONE',  ( 7.500000000000005329, -3.018576030000263533, 8.916666666666683838 ) ) ;
#11569=CARTESIAN_POINT ( 'NONE',  ( 10.49999999999999467, -13.50000000000000888, 9.250000000000063949 ) ) ;
#11589=CARTESIAN_POINT ( 'NONE',  ( -12.84999999999999964, -2.000000000000001776, 0.000000000000000000 ) ) ;
#11593=CARTESIAN_POINT ( 'NONE',  ( -7.710998176012597405, -11.54387914083317668, 8.114728912742389610 ) ) ;
#11594=CARTESIAN_POINT ( 'NONE',  ( -8.115139842999290920, -13.89206392873134099, 7.423524081915784834 ) ) ;
#11600=FILL_AREA_STYLE_COLOUR ( '', #22502 ) ;
#11610=CARTESIAN_POINT ( 'NONE',  ( -10.50000000000000888, 0.000000000000000000, 9.249999999999994671 ) ) ;
#11612=AXIS2_PLACEMENT_3D ( 'NONE', #11351, #20085, #5735 ) ;
#11619=CARTESIAN_POINT ( 'NONE',  ( 10.49999999999999467, -2.000000000000001776, 9.249999999999980460 ) ) ;
#11620=FACE_OUTER_BOUND ( 'NONE', #3431, .T. ) ;
#11621=PRODUCT_DEFINITION_FORMATION_WITH_SPECIFIED_SOURCE ( 'ANY', '', #18870, .NOT_KNOWN. ) ;
#11635=CARTESIAN_POINT ( 'NONE',  ( 8.697224362268011433, -12.50000000000002842, 6.250000000000061284 ) ) ;
#11637=ADVANCED_FACE ( 'NONE', ( #21341, #3224, #17438 ), #8506, .F. ) ;
#11662=ORIENTED_EDGE ( 'NONE', *, *, #7180, .T. ) ;
#11663=CIRCLE ( 'NONE', #12425, 2.549999999999997158 ) ;
#11676=DIRECTION ( 'NONE',  ( 1.000000000000000000, 1.910522504832140594E-31, -5.551115123125818447E-17 ) ) ;
#11678=LINE ( 'NONE', #13803, #6672 ) ;
#11684=DIRECTION ( 'NONE',  ( 0.000000000000000000, 3.469446951953618922E-15, 1.000000000000000000 ) ) ;
#11686=EDGE_LOOP ( 'NONE', ( #21607, #11215, #2442, #16568 ) ) ;
#11691=VERTEX_POINT ( 'NONE', #1446 ) ;
#11692=ORIENTED_EDGE ( 'NONE', *, *, #1501, .T. ) ;
#11699=CARTESIAN_POINT ( 'NONE',  ( -12.84999999999999964, 0.000000000000000000, 0.000000000000000000 ) ) ;
#11700=ORIENTED_EDGE ( 'NONE', *, *, #6745, .F. ) ;
#11707=CARTESIAN_POINT ( 'NONE',  ( -7.000000000000033751, -10.98142396999974579, 8.916666666666724694 ) ) ;
#11726=VERTEX_POINT ( 'NONE', #19795 ) ;
#11731=VERTEX_POINT ( 'NONE', #4010 ) ;
#11742=DIRECTION ( 'NONE',  ( -6.656013887802287108E-31, -1.000000000000000000, 3.469446951953609061E-15 ) ) ;
#11755=VERTEX_POINT ( 'NONE', #161 ) ;
#11762=CARTESIAN_POINT ( 'NONE',  ( -6.999999999999992006, -1.390227771353544473, 9.249999999999994671 ) ) ;
#11789=AXIS2_PLACEMENT_3D ( 'NONE', #11610, #9979, #4787 ) ;
#11790=LINE ( 'NONE', #15432, #21600 ) ;
#11806=CARTESIAN_POINT ( 'NONE',  ( -8.495599073428101278, -12.48424298295908130, 7.013360899078390887 ) ) ;
#11817=ORIENTED_EDGE ( 'NONE', *, *, #1042, .F. ) ;
#11826=DIRECTION ( 'NONE',  ( 0.000000000000000000, 0.000000000000000000, 1.000000000000000000 ) ) ;
#11859=DIRECTION ( 'NONE',  ( 0.000000000000000000, 0.000000000000000000, 1.000000000000000000 ) ) ;
#11866=( NAMED_UNIT ( * ) SI_UNIT ( $, .STERADIAN. ) SOLID_ANGLE_UNIT ( ) );
#11869=AXIS2_PLACEMENT_3D ( 'NONE', #9487, #13142, #2540 ) ;
#11875=CARTESIAN_POINT ( 'NONE',  ( 7.499999999999992895, -5.999999999999981348, 10.25000000000000888 ) ) ;
#11891=ORIENTED_EDGE ( 'NONE', *, *, #17135, .T. ) ;
#11896=ORIENTED_EDGE ( 'NONE', *, *, #6808, .F. ) ;
#11914=CARTESIAN_POINT ( 'NONE',  ( -8.113551354210013500, -12.41661007101923175, 7.426820295479667600 ) ) ;
#11915=LINE ( 'NONE', #13580, #4415 ) ;
#11926=ORIENTED_EDGE ( 'NONE', *, *, #19052, .T. ) ;
#11928=CIRCLE ( 'NONE', #4801, 6.000000000000000000 ) ;
#11940=DIRECTION ( 'NONE',  ( -1.454462294001240516E-30, -1.000000000000000000, 0.000000000000000000 ) ) ;
#11946=ADVANCED_FACE ( 'NONE', ( #13981 ), #7060, .T. ) ;
#11958=DIRECTION ( 'NONE',  ( 1.454462294001240516E-30, 1.000000000000000000, 0.000000000000000000 ) ) ;
#11960=PLANE ( 'NONE',  #22256 ) ;
#11963=ADVANCED_FACE ( 'NONE', ( #21527 ), #5024, .T. ) ;
#11968=CARTESIAN_POINT ( 'NONE',  ( -7.573440241539831419, -0.1138337924791395506, 7.421600184846377068 ) ) ;
#11974=EDGE_CURVE ( 'NONE', #1206, #9571, #1278, .T. ) ;
#11979=EDGE_CURVE ( 'NONE', #20776, #9332, #10281, .T. ) ;
#11999=CARTESIAN_POINT ( 'NONE',  ( -7.499999999999992895, -12.00000000000004263, 6.250000000000033751 ) ) ;
#12002=EDGE_CURVE ( 'NONE', #18123, #1546, #20688, .T. ) ;
#12007=ORIENTED_EDGE ( 'NONE', *, *, #17720, .F. ) ;
#12008=ORIENTED_EDGE ( 'NONE', *, *, #19412, .F. ) ;
#12017=CARTESIAN_POINT ( 'NONE',  ( -8.498922697886580835, -1.509195795641812499, 6.997949321565075209 ) ) ;
#12040=DIRECTION ( 'NONE',  ( -1.000000000000000000, 2.168404344971005170E-16, -1.203141491611682442E-30 ) ) ;
#12048=DIRECTION ( 'NONE',  ( 0.000000000000000000, 0.000000000000000000, 1.000000000000000000 ) ) ;
#12051=CARTESIAN_POINT ( 'NONE',  ( -7.629227790279464294, -1.952801550923857654, 8.369856247450591979 ) ) ;
#12064=LINE ( 'NONE', #6792, #15104 ) ;
#12073=CARTESIAN_POINT ( 'NONE',  ( 10.49999999999996803, -12.00000000000004796, 6.250000000000033751 ) ) ;
#12080=ORIENTED_EDGE ( 'NONE', *, *, #19043, .T. ) ;
#12115=CIRCLE ( 'NONE', #17775, 6.249999999999992006 ) ;
#12118=EDGE_LOOP ( 'NONE', ( #9095, #12292, #89, #7885 ) ) ;
#12119=CIRCLE ( 'NONE', #5747, 0.4999999999999995559 ) ;
#12186=DIRECTION ( 'NONE',  ( 0.000000000000000000, -6.938893903907237844E-15, -1.000000000000000000 ) ) ;
#12198=CARTESIAN_POINT ( 'NONE',  ( 7.518994333257404072, -2.258039616118832971, 8.837702940568432197 ) ) ;
#12199=DIRECTION ( 'NONE',  ( 1.000000000000000000, 6.224605580259554159E-31, -2.887593071917436153E-31 ) ) ;
#12203=LINE ( 'NONE', #10564, #4792 ) ;
#12219=CARTESIAN_POINT ( 'NONE',  ( -7.554637128289425796, -13.87985946887537558, 7.453047528892608575 ) ) ;
#12222=DIRECTION ( 'NONE',  ( 0.000000000000000000, 6.802837160693368935E-15, 1.000000000000000000 ) ) ;
#12239=DIRECTION ( 'NONE',  ( -9.121204216617949000E-31, -1.000000000000000000, 6.982962677686261977E-15 ) ) ;
#12245=EDGE_CURVE ( 'NONE', #8077, #3149, #20195, .T. ) ;
#12254=CARTESIAN_POINT ( 'NONE',  ( -8.954763739086851970, -12.50000000000002132, 6.678571428571506097 ) ) ;
#12276=CARTESIAN_POINT ( 'NONE',  ( -7.733764002503169088, -13.25269934883866263, 8.082002268151521562 ) ) ;
#12278=AXIS2_PLACEMENT_3D ( 'NONE', #12672, #12199, #6931 ) ;
#12281=CARTESIAN_POINT ( 'NONE',  ( -8.954763739086851970, -0.5000000000000004441, 6.678571428571422608 ) ) ;
#12283=DIRECTION ( 'NONE',  ( 1.454462294001240516E-30, 1.000000000000000000, 0.000000000000000000 ) ) ;
#12292=ORIENTED_EDGE ( 'NONE', *, *, #8505, .F. ) ;
#12299=AXIS2_PLACEMENT_3D ( 'NONE', #5860, #16884, #6202 ) ;
#12304=DIRECTION ( 'NONE',  ( 1.454462294001240516E-30, 1.000000000000000000, 0.000000000000000000 ) ) ;
#12310=CYLINDRICAL_SURFACE ( 'NONE', #9109, 0.4999999999999995559 ) ;
#12313=CARTESIAN_POINT ( 'NONE',  ( -8.204963667274123296, -0.08625821904939658114, 7.312308861538882709 ) ) ;
#12328=AXIS2_PLACEMENT_3D ( 'NONE', #10903, #8689, #1516 ) ;
#12335=EDGE_CURVE ( 'NONE', #17392, #10026, #14538, .T. ) ;
#12342=STYLED_ITEM ( 'NONE', ( #1264 ), #8352 ) ;
#12363=CARTESIAN_POINT ( 'NONE',  ( -12.84999999999999964, -12.00000000000002842, 5.750000000000018652 ) ) ;
#12365=DIRECTION ( 'NONE',  ( 0.000000000000000000, 0.8381404052084411305, -0.5454545454545505212 ) ) ;
#12366=CIRCLE ( 'NONE', #7492, 2.999999999999995559 ) ;
#12367=FACE_OUTER_BOUND ( 'NONE', #16828, .T. ) ;
#12368=CARTESIAN_POINT ( 'NONE',  ( 12.84999999999997300, 0.000000000000000000, -2.549999999999986944 ) ) ;
#12369=CARTESIAN_POINT ( 'NONE',  ( -7.271441198316176191, -0.2709289393878913099, 8.039702399269740951 ) ) ;
#12371=FACE_OUTER_BOUND ( 'NONE', #9766, .T. ) ;
#12388=EDGE_CURVE ( 'NONE', #18942, #10463, #8431, .T. ) ;
#12399=CARTESIAN_POINT ( 'NONE',  ( -12.84999999999999964, -2.000000000000001776, 5.750000000000005329 ) ) ;
#12402=DIRECTION ( 'NONE',  ( 2.168404344971005170E-16, 1.000000000000000000, -8.696324126752285467E-47 ) ) ;
#12414=DIRECTION ( 'NONE',  ( 1.000000000000000000, 4.252453317207022018E-31, -5.551115123125818447E-17 ) ) ;
#12422=VERTEX_POINT ( 'NONE', #15222 ) ;
#12425=AXIS2_PLACEMENT_3D ( 'NONE', #19178, #10348, #20952 ) ;
#12430=DIRECTION ( 'NONE',  ( -9.121204216617949000E-31, -1.000000000000000000, 6.982962677686261977E-15 ) ) ;
#12453=EDGE_LOOP ( 'NONE', ( #19701, #8961, #22471, #21286, #9363, #16083 ) ) ;
#12460=CARTESIAN_POINT ( 'NONE',  ( -7.332081355611494544, -13.77321347121581319, 7.890992604157061052 ) ) ;
#12467=ORIENTED_EDGE ( 'NONE', *, *, #11241, .F. ) ;
#12470=ORIENTED_EDGE ( 'NONE', *, *, #15156, .T. ) ;
#12481=CARTESIAN_POINT ( 'NONE',  ( -8.160037397871438003, -0.008793114504473772963, 6.662331851011921380 ) ) ;
#12494=CARTESIAN_POINT ( 'NONE',  ( -12.84999999999998721, -12.50000000000002842, 5.750000000000060396 ) ) ;
#12497=EDGE_LOOP ( 'NONE', ( #19568, #3916, #3585, #9185 ) ) ;
#12515=DIRECTION ( 'NONE',  ( -1.445602896647339163E-16, 1.000000000000000000, 0.000000000000000000 ) ) ;
#12522=FACE_OUTER_BOUND ( 'NONE', #14056, .T. ) ;
#12526=CARTESIAN_POINT ( 'NONE',  ( -7.884991313526885648, -1.682691736113209213, 7.773664271103597478 ) ) ;
#12533=DIRECTION ( 'NONE',  ( 0.5150787536377134934, 0.000000000000000000, 0.8571428571428567622 ) ) ;
#12540=EDGE_LOOP ( 'NONE', ( #11692, #19282, #11401, #18389, #10516, #23090 ) ) ;
#12545=CARTESIAN_POINT ( 'NONE',  ( 7.909386411297023578, -0.6370970679665967085, 7.731447622712498635 ) ) ;
#12551=DIRECTION ( 'NONE',  ( 1.000000000000000000, 6.224605580259554159E-31, -2.887593071917436153E-31 ) ) ;
#12554=ADVANCED_FACE ( 'NONE', ( #4869 ), #930, .T. ) ;
#12557=DIRECTION ( 'NONE',  ( 0.000000000000000000, 0.000000000000000000, -1.000000000000000000 ) ) ;
#12564=DIRECTION ( 'NONE',  ( 1.454462294001240516E-30, 1.000000000000000000, 0.000000000000000000 ) ) ;
#12602=CARTESIAN_POINT ( 'NONE',  ( 7.725871784772684769, -12.18565941508499861, 8.100883686805255834 ) ) ;
#12610=DIRECTION ( 'NONE',  ( 1.000000000000000000, 1.910522504832140594E-31, -5.551115123125818447E-17 ) ) ;
#12613=CARTESIAN_POINT ( 'NONE',  ( 12.84999999999997300, -14.00000000000007105, 5.551115123125782702E-14 ) ) ;
#12615=CARTESIAN_POINT ( 'NONE',  ( 7.856071383949647213, -0.04768060911160624388, 7.015054140272313887 ) ) ;
#12617=( GEOMETRIC_REPRESENTATION_CONTEXT ( 3 ) GLOBAL_UNCERTAINTY_ASSIGNED_CONTEXT ( ( #8378 ) ) GLOBAL_UNIT_ASSIGNED_CONTEXT ( ( #9637, #6116, #11866 ) ) REPRESENTATION_CONTEXT ( 'NONE', 'WORKASPACE' ) );
#12623=ORIENTED_EDGE ( 'NONE', *, *, #17112, .T. ) ;
#12633=CARTESIAN_POINT ( 'NONE',  ( -6.999999999999992006, -2.645898033750305522, 9.250000000000021316 ) ) ;
#12644=AXIS2_PLACEMENT_3D ( 'NONE', #3160, #3497, #10669 ) ;
#12650=EDGE_LOOP ( 'NONE', ( #12467, #19956 ) ) ;
#12655=DIRECTION ( 'NONE',  ( -1.454462294001240516E-30, -1.000000000000000000, 0.000000000000000000 ) ) ;
#12660=FACE_OUTER_BOUND ( 'NONE', #19980, .T. ) ;
#12665=CARTESIAN_POINT ( 'NONE',  ( -7.162073728446612719, -2.365283217609512434, 7.945145523438274182 ) ) ;
#12672=CARTESIAN_POINT ( 'NONE',  ( 12.84999999999998721, -1.500000000000004885, -5.749999999999976907 ) ) ;
#12677=LINE ( 'NONE', #15965, #19432 ) ;
#12686=ORIENTED_EDGE ( 'NONE', *, *, #5389, .F. ) ;
#12687=APPLICATION_CONTEXT ( 'automotive_design' ) ;
#12691=CARTESIAN_POINT ( 'NONE',  ( 6.999999999999978684, -10.98142396999974757, 8.916666666666712260 ) ) ;
#12702=CYLINDRICAL_SURFACE ( 'NONE', #16412, 0.4999999999999995559 ) ;
#12711=CIRCLE ( 'NONE', #4423, 0.4999999999999995559 ) ;
#12720=CARTESIAN_POINT ( 'NONE',  ( 8.697224362267983011, 0.000000000000000000, 6.249999999999977796 ) ) ;
#12721=CARTESIAN_POINT ( 'NONE',  ( 7.161440864725792999, -11.61224748569070009, 7.973376427817330914 ) ) ;
#12734=DIRECTION ( 'NONE',  ( 0.000000000000000000, 0.000000000000000000, 1.000000000000000000 ) ) ;
#12736=CARTESIAN_POINT ( 'NONE',  ( 7.500000000000008882, -0.9711575687493221309, 9.522727272727294690 ) ) ;
#12742=AXIS2_PLACEMENT_3D ( 'NONE', #18073, #8548, #23144 ) ;
#12764=DIRECTION ( 'NONE',  ( -2.168404344971017743E-16, -1.000000000000000000, 6.982962677686261977E-15 ) ) ;
#12766=ORIENTED_EDGE ( 'NONE', *, *, #14485, .F. ) ;
#12774=VERTEX_POINT ( 'NONE', #18060 ) ;
#12782=CARTESIAN_POINT ( 'NONE',  ( 7.884991313526920287, -12.31730826388680633, 7.773664271103689849 ) ) ;
#12784=AXIS2_PLACEMENT_3D ( 'NONE', #8081, #22786, #6560 ) ;
#12785=CARTESIAN_POINT ( 'NONE',  ( -6.999999995230847816, -13.21736471697163395, 9.233045673661568031 ) ) ;
#12787=DIRECTION ( 'NONE',  ( -2.168404344971017743E-16, -1.000000000000000000, 6.982962677686261977E-15 ) ) ;
#12789=CARTESIAN_POINT ( 'NONE',  ( -7.499999999999992895, -8.000000000000044409, 6.250000000000005329 ) ) ;
#12794=EDGE_CURVE ( 'NONE', #3149, #11755, #13311, .T. ) ;
#12834=DIRECTION ( 'NONE',  ( 0.000000000000000000, 0.000000000000000000, 1.000000000000000000 ) ) ;
#12836=CARTESIAN_POINT ( 'NONE',  ( -12.84999999999999964, -0.5000000000000004441, 0.000000000000000000 ) ) ;
#12843=DIRECTION ( 'NONE',  ( 0.000000000000000000, 0.000000000000000000, -1.000000000000000000 ) ) ;
#12858=EDGE_LOOP ( 'NONE', ( #6439, #14885, #10338, #3760 ) ) ;
#12872=VECTOR ( 'NONE', #17726, 1000.000000000000000 ) ;
#12891=ORIENTED_EDGE ( 'NONE', *, *, #21749, .F. ) ;
#12904=CYLINDRICAL_SURFACE ( 'NONE', #7930, 6.249999999999992006 ) ;
#12908=CIRCLE ( 'NONE', #18172, 5.749999999999992006 ) ;
#12910=CARTESIAN_POINT ( 'NONE',  ( -8.079084010241013303, -2.020344040167372679, 6.665520415301724455 ) ) ;
#12911=PLANE ( 'NONE',  #12299 ) ;
#12916=AXIS2_PLACEMENT_3D ( 'NONE', #22667, #17350, #11477 ) ;
#12917=CIRCLE ( 'NONE', #18203, 0.4999999999999999445 ) ;
#12922=ORIENTED_EDGE ( 'NONE', *, *, #6624, .T. ) ;
#12924=FACE_OUTER_BOUND ( 'NONE', #10362, .T. ) ;
#12928=DIRECTION ( 'NONE',  ( 1.000000000000000000, 1.910522504832140594E-31, -5.551115123125818447E-17 ) ) ;
#12933=CARTESIAN_POINT ( 'NONE',  ( 6.999999999999982236, -13.02884243125068942, 9.522727272727369296 ) ) ;
#12941=LINE ( 'NONE', #11170, #2472 ) ;
#12943=B_SPLINE_CURVE_WITH_KNOTS ( 'NONE', 3,
 ( #4001, #20012, #12952, #21895, #5893, #5446, #7658, #19905, #149, #21561, #20252, #11182, #7325, #12720 ),
 .UNSPECIFIED., .F., .F.,
 ( 4, 2, 2, 2, 2, 2, 4 ),
 ( 0.000000000000000000, 0.001000930383652479062, 0.001501395575478720653, 0.002001860767304962461, 0.002502325959131204269, 0.003002791150957445643, 0.004003721534609925789 ),
 .UNSPECIFIED. ) ;
#12948=ORIENTED_EDGE ( 'NONE', *, *, #9248, .T. ) ;
#12952=CARTESIAN_POINT ( 'NONE',  ( 7.028413389564965641, -0.6300521812368736763, 8.946655872546013910 ) ) ;
#12954=CARTESIAN_POINT ( 'NONE',  ( 7.602880770961806256, -11.99349919129478614, 8.461619612152116332 ) ) ;
#12957=DIRECTION ( 'NONE',  ( 1.454462294001240516E-30, 1.000000000000000000, 0.000000000000000000 ) ) ;
#12958=DIRECTION ( 'NONE',  ( 5.551115123125790098E-17, 6.982962677686276177E-15, 1.000000000000000000 ) ) ;
#12959=EDGE_CURVE ( 'NONE', #1546, #20509, #19680, .T. ) ;
#12972=EDGE_CURVE ( 'NONE', #17687, #12422, #14032, .T. ) ;
#12974=CARTESIAN_POINT ( 'NONE',  ( 7.742458795615140055, -0.7399311281350806624, 8.061568688625849077 ) ) ;
#12975=EDGE_CURVE ( 'NONE', #15314, #2644, #6534, .T. ) ;
#12984=ORIENTED_EDGE ( 'NONE', *, *, #6807, .F. ) ;
#12992=FACE_OUTER_BOUND ( 'NONE', #12497, .T. ) ;
#13003=DIRECTION ( 'NONE',  ( 2.797982890317280824E-17, 0.6666666666666667407, -0.7453559924999300090 ) ) ;
#13007=ORIENTED_EDGE ( 'NONE', *, *, #5862, .F. ) ;
#13024=FACE_OUTER_BOUND ( 'NONE', #10660, .T. ) ;
#13038=CIRCLE ( 'NONE', #5902, 2.999999999999995559 ) ;
#13049=CARTESIAN_POINT ( 'NONE',  ( 8.697224362267983011, 0.000000000000000000, 6.249999999999977796 ) ) ;
#13050=CARTESIAN_POINT ( 'NONE',  ( 7.345446946324464044, -13.78184793132693819, 7.860330092054047313 ) ) ;
#13055=DIRECTION ( 'NONE',  ( -6.656013887802287108E-31, -1.000000000000000000, 3.469446951953609061E-15 ) ) ;
#13078=DIRECTION ( 'NONE',  ( 5.551115123125818447E-17, 6.982962677686276177E-15, 1.000000000000000000 ) ) ;
#13085=CARTESIAN_POINT ( 'NONE',  ( 8.178874953434444706, -0.007851515978188753839, 6.644730819939002053 ) ) ;
#13089=ORIENTED_EDGE ( 'NONE', *, *, #12972, .F. ) ;
#13090=ADVANCED_FACE ( 'NONE', ( #5673 ), #5020, .T. ) ;
#13095=ORIENTED_EDGE ( 'NONE', *, *, #10928, .F. ) ;
#13130=ORIENTED_EDGE ( 'NONE', *, *, #7676, .F. ) ;
#13141=DIRECTION ( 'NONE',  ( 1.000000000000000000, 1.910522504832140594E-31, -5.551115123125818447E-17 ) ) ;
#13142=DIRECTION ( 'NONE',  ( 0.8571428571428567622, 8.935192059122191449E-16, -0.5150787536377136044 ) ) ;
#13143=CARTESIAN_POINT ( 'NONE',  ( -6.999999999999992006, -13.02884243125068409, 9.522727272727356862 ) ) ;
#13169=LINE ( 'NONE', #15032, #7946 ) ;
#13183=ORIENTED_EDGE ( 'NONE', *, *, #4970, .F. ) ;
#13189=DIRECTION ( 'NONE',  ( 0.000000000000000000, -0.8381404052084435730, -0.5454545454545466354 ) ) ;
#13193=DIRECTION ( 'NONE',  ( -1.000000000000000000, -4.252453317207022018E-31, 5.551115123125818447E-17 ) ) ;
#13196=CARTESIAN_POINT ( 'NONE',  ( -8.697224362267997222, -1.999999999999998224, 6.249999999999977796 ) ) ;
#13204=ORIENTED_EDGE ( 'NONE', *, *, #8358, .F. ) ;
#13237=AXIS2_PLACEMENT_3D ( 'NONE', #11699, #17101, #20892 ) ;
#13247=FACE_OUTER_BOUND ( 'NONE', #22072, .T. ) ;
#13249=CARTESIAN_POINT ( 'NONE',  ( -6.999999991915196951, -11.17450167042466092, 8.700799235122007147 ) ) ;
#13251=CARTESIAN_POINT ( 'NONE',  ( -8.233775472210666635, -13.45629277298747262, 7.279685395985863394 ) ) ;
#13254=LINE ( 'NONE', #22320, #7660 ) ;
#13256=DIRECTION ( 'NONE',  ( 0.000000000000000000, 0.000000000000000000, 1.000000000000000000 ) ) ;
#13263=ORIENTED_EDGE ( 'NONE', *, *, #8505, .T. ) ;
#13275=DIRECTION ( 'NONE',  ( 0.000000000000000000, 0.000000000000000000, -1.000000000000000000 ) ) ;
#13277=DIRECTION ( 'NONE',  ( 9.121204216617949000E-31, 1.000000000000000000, -6.982962677686261977E-15 ) ) ;
#13297=VECTOR ( 'NONE', #4435, 1000.000000000000000 ) ;
#13311=CIRCLE ( 'NONE', #8052, 0.4999999999999995559 ) ;
#13320=CARTESIAN_POINT ( 'NONE',  ( 10.49999999999999467, -12.50000000000000711, 9.250000000000063949 ) ) ;
#13322=DIRECTION ( 'NONE',  ( 0.000000000000000000, -6.938893903907237844E-15, -1.000000000000000000 ) ) ;
#13326=ORIENTED_EDGE ( 'NONE', *, *, #3610, .T. ) ;
#13328=UNCERTAINTY_MEASURE_WITH_UNIT (LENGTH_MEASURE( 1.000000000000000082E-05 ), #22674, 'distance_accuracy_value', 'NONE');
#13335=DIRECTION ( 'NONE',  ( 6.656013887802287108E-31, 1.000000000000000000, -3.469446951953609061E-15 ) ) ;
#13343=CARTESIAN_POINT ( 'NONE',  ( -8.697224362268023867, -12.50000000000002842, 6.250000000000088818 ) ) ;
#13350=DIRECTION ( 'NONE',  ( 1.431475090352998897E-31, -3.469446951953609061E-15, -1.000000000000000000 ) ) ;
#13370=CARTESIAN_POINT ( 'NONE',  ( -8.181569977154559581, -11.86479625201650556, 7.340676138759481439 ) ) ;
#13371=CARTESIAN_POINT ( 'NONE',  ( -7.796097383573772355, -13.30002726899557075, 7.943830786858237403 ) ) ;
#13387=FACE_OUTER_BOUND ( 'NONE', #21702, .T. ) ;
#13388=CARTESIAN_POINT ( 'NONE',  ( -7.500000000000020428, -1.999999999999991340, 9.250000000000008882 ) ) ;
#13397=CARTESIAN_POINT ( 'NONE',  ( 8.954763739086850194, -14.00000000000004263, 6.678571428571495439 ) ) ;
#13412=VERTEX_POINT ( 'NONE', #2096 ) ;
#13420=ORIENTED_EDGE ( 'NONE', *, *, #7109, .T. ) ;
#13426=DIRECTION ( 'NONE',  ( 0.000000000000000000, 0.000000000000000000, -1.000000000000000000 ) ) ;
#13428=CARTESIAN_POINT ( 'NONE',  ( -12.84999999999999964, -0.5000000000000038858, 6.250000000000033751 ) ) ;
#13439=ADVANCED_FACE ( 'NONE', ( #9404 ), #3978, .T. ) ;
#13455=CARTESIAN_POINT ( 'NONE',  ( -8.954763739086814667, -1.499999999999987566, 6.678571428571395074 ) ) ;
#13463=DIRECTION ( 'NONE',  ( 6.656013887802287108E-31, 1.000000000000000000, -3.469446951953609061E-15 ) ) ;
#13465=CARTESIAN_POINT ( 'NONE',  ( -7.499999999999992895, -5.999999999999987566, 6.249999999999992006 ) ) ;
#13472=EDGE_CURVE ( 'NONE', #2644, #10463, #2221, .T. ) ;
#13473=CIRCLE ( 'NONE', #19868, 2.549999999999997158 ) ;
#13474=EDGE_LOOP ( 'NONE', ( #11209, #978, #8177, #2491 ) ) ;
#13476=CIRCLE ( 'NONE', #7846, 0.4999999999999995559 ) ;
#13481=DIRECTION ( 'NONE',  ( 0.000000000000000000, 6.802837160693368935E-15, 1.000000000000000000 ) ) ;
#13483=ORIENTED_EDGE ( 'NONE', *, *, #208, .F. ) ;
#13488=DIRECTION ( 'NONE',  ( 2.168404344971008868E-16, 1.000000000000000000, -8.890457814381136359E-15 ) ) ;
#13491=CIRCLE ( 'NONE', #12784, 0.4999999999999999445 ) ;
#13504=LINE ( 'NONE', #15020, #21888 ) ;
#13507=ORIENTED_EDGE ( 'NONE', *, *, #11419, .F. ) ;
#13518=CARTESIAN_POINT ( 'NONE',  ( 8.954763739086848418, -13.50000000000004441, 6.678571428571493662 ) ) ;
#13525=DIRECTION ( 'NONE',  ( 0.000000000000000000, 6.802837160693368935E-15, 1.000000000000000000 ) ) ;
#13531=ORIENTED_EDGE ( 'NONE', *, *, #14443, .T. ) ;
#13543=LINE ( 'NONE', #13428, #22999 ) ;
#13556=VERTEX_POINT ( 'NONE', #579 ) ;
#13558=ORIENTED_EDGE ( 'NONE', *, *, #1636, .T. ) ;
#13570=EDGE_CURVE ( 'NONE', #18328, #138, #7879, .T. ) ;
#13573=CARTESIAN_POINT ( 'NONE',  ( 7.161440864725725497, -2.387752514309381180, 7.973376427817429501 ) ) ;
#13580=CARTESIAN_POINT ( 'NONE',  ( -12.84999999999999964, -2.000000000000001776, -2.549999999999997158 ) ) ;
#13596=DIRECTION ( 'NONE',  ( -1.000000000000000000, -6.224605580259554159E-31, 2.887593071917436153E-31 ) ) ;
#13606=DIRECTION ( 'NONE',  ( 4.313844246609350428E-33, 6.982962677686276966E-15, 1.000000000000000000 ) ) ;
#13620=ORIENTED_EDGE ( 'NONE', *, *, #10825, .T. ) ;
#13622=ORIENTED_EDGE ( 'NONE', *, *, #11974, .T. ) ;
#13631=CARTESIAN_POINT ( 'NONE',  ( -7.479729963940282111, -0.8034648269414370603, 9.265052153041423821 ) ) ;
#13633=VECTOR ( 'NONE', #532, 1000.000000000000000 ) ;
#13634=CIRCLE ( 'NONE', #7987, 0.4999999999999995559 ) ;
#13648=CIRCLE ( 'NONE', #20419, 6.000000000000000000 ) ;
#13657=DIRECTION ( 'NONE',  ( -1.000000000000000000, 2.168404344971005170E-16, -1.203141491611682442E-30 ) ) ;
#13660=AXIS2_PLACEMENT_3D ( 'NONE', #5277, #4504, #6930 ) ;
#13674=VERTEX_POINT ( 'NONE', #12399 ) ;
#13683=EDGE_CURVE ( 'NONE', #3406, #12422, #20660, .T. ) ;
#13687=CARTESIAN_POINT ( 'NONE',  ( -7.263517083688543430, -2.279413854694210428, 7.724990489865457555 ) ) ;
#13691=CARTESIAN_POINT ( 'NONE',  ( 8.181569977154431683, -2.135203747983557498, 7.340676138759591574 ) ) ;
#13696=DIRECTION ( 'NONE',  ( -1.000000000000000000, -1.910522504832140594E-31, 5.551115123125818447E-17 ) ) ;
#13712=CARTESIAN_POINT ( 'NONE',  ( -12.85000000000001386, -12.00000000000006928, 4.163336342344337027E-14 ) ) ;
#13737=DIRECTION ( 'NONE',  ( 1.000000000000000000, 4.252453317207022894E-31, -5.551115123125818447E-17 ) ) ;
#13741=DIRECTION ( 'NONE',  ( -5.551115123125761132E-17, 1.577721810442025713E-30, -1.000000000000000000 ) ) ;
#13744=DIRECTION ( 'NONE',  ( -1.000000000000000000, -1.910522504832140594E-31, 5.551115123125818447E-17 ) ) ;
#13749=CARTESIAN_POINT ( 'NONE',  ( -8.510464245293276164, -0.5071972189927809183, 6.988717072693961363 ) ) ;
#13769=EDGE_LOOP ( 'NONE', ( #3716, #22037, #19777, #16662 ) ) ;
#13770=CARTESIAN_POINT ( 'NONE',  ( -12.84999999999999964, -0.5000000000000038858, 6.250000000000033751 ) ) ;
#13778=CARTESIAN_POINT ( 'NONE',  ( 12.84999999999997300, -0.5000000000000004441, 5.750000000000018652 ) ) ;
#13803=CARTESIAN_POINT ( 'NONE',  ( -12.85000000000005649, -13.50000000000011191, -6.249999999999921840 ) ) ;
#13806=DIRECTION ( 'NONE',  ( 9.121204216617949000E-31, 1.000000000000000000, -6.982962677686261977E-15 ) ) ;
#13819=VERTEX_POINT ( 'NONE', #642 ) ;
#13823=CIRCLE ( 'NONE', #10809, 2.549999999999997158 ) ;
#13849=LINE ( 'NONE', #15721, #10981 ) ;
#13858=TOROIDAL_SURFACE ( 'NONE', #1447, 3.500000000000000000, 0.5000000000000000000 ) ;
#13864=LINE ( 'NONE', #12073, #17190 ) ;
#13881=DIRECTION ( 'NONE',  ( 1.000000000000000000, 4.252453317207022018E-31, -5.551115123125818447E-17 ) ) ;
#13886=DIRECTION ( 'NONE',  ( -1.000000000000000000, -4.252453317207022018E-31, 5.551115123125818447E-17 ) ) ;
#13902=ORIENTED_EDGE ( 'NONE', *, *, #12388, .F. ) ;
#13903=ORIENTED_EDGE ( 'NONE', *, *, #10928, .T. ) ;
#13904=DIRECTION ( 'NONE',  ( -2.168404344971017743E-16, 1.000000000000000000, 1.287063703585503763E-46 ) ) ;
#13924=ORIENTED_EDGE ( 'NONE', *, *, #1392, .T. ) ;
#13930=DIRECTION ( 'NONE',  ( -9.121204216617949000E-31, -1.000000000000000000, 6.982962677686261977E-15 ) ) ;
#13932=CARTESIAN_POINT ( 'NONE',  ( -6.999999999999992006, -5.999999999999987566, 6.250000000000005329 ) ) ;
#13941=PLANE ( 'NONE',  #16844 ) ;
#13943=CARTESIAN_POINT ( 'NONE',  ( -7.595478965369684587, -2.023942297479878416, 8.489833260407415594 ) ) ;
#13947=CARTESIAN_POINT ( 'NONE',  ( 6.999999999999978684, -12.60977222864647196, 9.250000000000092371 ) ) ;
#13955=DIRECTION ( 'NONE',  ( 1.000000000000000000, 6.224605580259554159E-31, -2.887593071917436153E-31 ) ) ;
#13958=CARTESIAN_POINT ( 'NONE',  ( 7.733764002503170865, -0.7473006511613611291, 8.082002268151491364 ) ) ;
#13972=CARTESIAN_POINT ( 'NONE',  ( 7.499999999999978684, -2.645898033750298417, 9.250000000000021316 ) ) ;
#13981=FACE_OUTER_BOUND ( 'NONE', #10193, .T. ) ;
#14009=VECTOR ( 'NONE', #12958, 1000.000000000000000 ) ;
#14021=DIRECTION ( 'NONE',  ( -2.887593071917436153E-31, -7.888609052210128564E-31, 1.000000000000000000 ) ) ;
#14030=CARTESIAN_POINT ( 'NONE',  ( 7.786490775660123376, -13.29349257805251305, 7.963863235126093620 ) ) ;
#14031=AXIS2_PLACEMENT_3D ( 'NONE', #17394, #22585, #22477 ) ;
#14032=CIRCLE ( 'NONE', #14405, 0.4999999999999998335 ) ;
#14040=CARTESIAN_POINT ( 'NONE',  ( -7.955953741309951255, -12.35582749618196274, 7.654083333123914201 ) ) ;
#14048=VECTOR ( 'NONE', #12928, 1000.000000000000000 ) ;
#14054=DIRECTION ( 'NONE',  ( 1.454462294001240516E-30, 1.000000000000000000, 0.000000000000000000 ) ) ;
#14056=EDGE_LOOP ( 'NONE', ( #16921, #21146, #6012, #10512 ) ) ;
#14060=DIRECTION ( 'NONE',  ( 0.000000000000000000, -7.888609052210128564E-31, 1.000000000000000000 ) ) ;
#14074=CARTESIAN_POINT ( 'NONE',  ( 8.697224362267983011, -0.5000000000000004441, 6.250000000000061284 ) ) ;
#14087=DIRECTION ( 'NONE',  ( 9.121204216617949000E-31, 1.000000000000000000, -6.982962677686261977E-15 ) ) ;
#14089=CARTESIAN_POINT ( 'NONE',  ( -7.282868595548795732, -0.2617430505220332271, 8.010178330700856719 ) ) ;
#14095=CARTESIAN_POINT ( 'NONE',  ( 7.629227790279506927, -1.952801550923872309, 8.369856247450629283 ) ) ;
#14109=EDGE_CURVE ( 'NONE', #9571, #18328, #9738, .T. ) ;
#14112=DIRECTION ( 'NONE',  ( -1.000000000000000000, -2.891205793294682764E-16, 0.000000000000000000 ) ) ;
#14118=CARTESIAN_POINT ( 'NONE',  ( 7.499999999999992895, -5.999999999999981348, 6.250000000000005329 ) ) ;
#14121=CARTESIAN_POINT ( 'NONE',  ( 7.835522544085462116, -2.050824327339876074, 6.894286109559123688 ) ) ;
#14123=DIRECTION ( 'NONE',  ( 1.454462294001240516E-30, 1.000000000000000000, 0.000000000000000000 ) ) ;
#14133=ADVANCED_FACE ( 'NONE', ( #18137 ), #22012, .T. ) ;
#14148=DIRECTION ( 'NONE',  ( 0.000000000000000000, 0.000000000000000000, 1.000000000000000000 ) ) ;
#14152=DIRECTION ( 'NONE',  ( -9.121204216617949000E-31, -1.000000000000000000, 6.982962677686261977E-15 ) ) ;
#14169=AXIS2_PLACEMENT_3D ( 'NONE', #13465, #22636, #11684 ) ;
#14171=CARTESIAN_POINT ( 'NONE',  ( -12.84999999999999964, -0.5000000000000004441, 0.000000000000000000 ) ) ;
#14178=VECTOR ( 'NONE', #7283, 1000.000000000000000 ) ;
#14179=CARTESIAN_POINT ( 'NONE',  ( -12.85000000000002807, -13.50000000000003020, 6.250000000000033751 ) ) ;
#14182=DIRECTION ( 'NONE',  ( -1.454462294001240516E-30, -1.000000000000000000, -0.000000000000000000 ) ) ;
#14188=CARTESIAN_POINT ( 'NONE',  ( -8.495599073428085291, -1.515757017040946009, 7.013360899078306510 ) ) ;
#14197=EDGE_CURVE ( 'NONE', #21322, #21919, #11283, .T. ) ;
#14205=EDGE_CURVE ( 'NONE', #18123, #19164, #14662, .T. ) ;
#14208=CARTESIAN_POINT ( 'NONE',  ( 7.499999999999977796, -1.223704156646852281, 9.030675447288961877 ) ) ;
#14212=CARTESIAN_POINT ( 'NONE',  ( -10.49999999999998224, -14.00000000000003020, 5.750000000000032863 ) ) ;
#14224=VECTOR ( 'NONE', #14957, 1000.000000000000000 ) ;
#14239=CARTESIAN_POINT ( 'NONE',  ( -7.835312244870005216, -13.94896639302768371, 7.041165740960562580 ) ) ;
#14242=CARTESIAN_POINT ( 'NONE',  ( 8.260108127873506234, -2.109168607890740788, 7.249251683976269511 ) ) ;
#14261=CARTESIAN_POINT ( 'NONE',  ( 7.500000000000007105, -11.35410196624971491, 9.250000000000014211 ) ) ;
#14263=FACE_OUTER_BOUND ( 'NONE', #31, .T. ) ;
#14267=CARTESIAN_POINT ( 'NONE',  ( -10.49999999999996803, -1.500000000000001332, 9.250000000000008882 ) ) ;
#14282=ORIENTED_EDGE ( 'NONE', *, *, #13472, .F. ) ;
#14291=EDGE_CURVE ( 'NONE', #7030, #9040, #20705, .T. ) ;
#14295=CARTESIAN_POINT ( 'NONE',  ( -7.500000000000034639, -12.77629584335315727, 9.030675447289006286 ) ) ;
#14296=DIRECTION ( 'NONE',  ( -5.273559366969500667E-15, -6.938893903907237055E-15, -1.000000000000000000 ) ) ;
#14305=CARTESIAN_POINT ( 'NONE',  ( -8.391189084741213833, -1.526797151860788349, 7.111621047081270852 ) ) ;
#14310=EDGE_LOOP ( 'NONE', ( #5521, #19188, #16630, #420 ) ) ;
#14321=CARTESIAN_POINT ( 'NONE',  ( 10.49999999999999467, -5.999999999999974243, 9.250000000000008882 ) ) ;
#14322=DIRECTION ( 'NONE',  ( -6.656013887802287108E-31, -1.000000000000000000, 3.469446951953609061E-15 ) ) ;
#14339=CARTESIAN_POINT ( 'NONE',  ( 7.491585531133591047, -11.85620892266378235, 7.320610673787135703 ) ) ;
#14348=CARTESIAN_POINT ( 'NONE',  ( -12.84999999999999964, -13.50000000000003020, 5.750000000000032863 ) ) ;
#14362=EDGE_CURVE ( 'NONE', #18328, #6218, #7913, .T. ) ;
#14363=ORIENTED_EDGE ( 'NONE', *, *, #17473, .T. ) ;
#14368=CARTESIAN_POINT ( 'NONE',  ( 7.500000000000008882, -10.98142396999974224, 8.916666666666674956 ) ) ;
#14371=CARTESIAN_POINT ( 'NONE',  ( 10.50000000000000888, -1.500000000000001332, 9.250000000000008882 ) ) ;
#14372=CARTESIAN_POINT ( 'NONE',  ( 12.84999999999997300, -12.50000000000006928, 5.551115123125782702E-14 ) ) ;
#14405=AXIS2_PLACEMENT_3D ( 'NONE', #17791, #20976, #12365 ) ;
#14428=ORIENTED_EDGE ( 'NONE', *, *, #17610, .T. ) ;
#14429=ORIENTED_EDGE ( 'NONE', *, *, #22600, .T. ) ;
#14431=EDGE_CURVE ( 'NONE', #6724, #16375, #18477, .T. ) ;
#14434=CIRCLE ( 'NONE', #12916, 4.500000000000000888 ) ;
#14435=ADVANCED_FACE ( 'NONE', ( #6714 ), #10128, .T. ) ;
#14443=EDGE_CURVE ( 'NONE', #9710, #17392, #11294, .T. ) ;
#14452=TOROIDAL_SURFACE ( 'NONE', #6563, 3.500000000000000000, 0.5000000000000000000 ) ;
#14456=CARTESIAN_POINT ( 'NONE',  ( 10.49999999999999467, -8.000000000000031974, 9.250000000000021316 ) ) ;
#14470=FACE_OUTER_BOUND ( 'NONE', #15746, .T. ) ;
#14472=CARTESIAN_POINT ( 'NONE',  ( -6.999999999999993783, -13.21292803502077184, 9.239863038076370216 ) ) ;
#14484=VERTEX_POINT ( 'NONE', #8479 ) ;
#14485=EDGE_CURVE ( 'NONE', #2116, #9302, #11663, .T. ) ;
#14486=ORIENTED_EDGE ( 'NONE', *, *, #5634, .F. ) ;
#14489=EDGE_CURVE ( 'NONE', #9370, #20776, #15758, .T. ) ;
#14492=CARTESIAN_POINT ( 'NONE',  ( -8.565230440156030411, -12.00000000000004441, 6.320505311736962284 ) ) ;
#14494=DIRECTION ( 'NONE',  ( -9.121204216617949000E-31, -1.000000000000000000, 6.982962677686261977E-15 ) ) ;
#14498=CARTESIAN_POINT ( 'NONE',  ( -8.697224362268011433, -1.499999999999984013, 6.250000000000005329 ) ) ;
#14499=FACE_OUTER_BOUND ( 'NONE', #17569, .T. ) ;
#14505=ORIENTED_EDGE ( 'NONE', *, *, #8411, .F. ) ;
#14527=EDGE_LOOP ( 'NONE', ( #2499, #20533, #5347, #7827, #1809, #3581 ) ) ;
#14530=VERTEX_POINT ( 'NONE', #10473 ) ;
#14537=ORIENTED_EDGE ( 'NONE', *, *, #18861, .F. ) ;
#14538=LINE ( 'NONE', #94, #15912 ) ;
#14545=CARTESIAN_POINT ( 'NONE',  ( 8.495599073428115489, -12.48424298295908130, 7.013360899078397992 ) ) ;
#14551=DIRECTION ( 'NONE',  ( 9.121204216617949000E-31, 1.000000000000000000, -6.982962677686261977E-15 ) ) ;
#14554=CIRCLE ( 'NONE', #22847, 3.499999999999995115 ) ;
#14566=CIRCLE ( 'NONE', #2156, 2.999999999999995559 ) ;
#14568=CARTESIAN_POINT ( 'NONE',  ( -12.84999999999999964, -2.011595308313580664E-30, 2.549999999999997158 ) ) ;
#14581=CARTESIAN_POINT ( 'NONE',  ( 7.168696526429616966, -13.62622308581068253, 8.340670630249162443 ) ) ;
#14582=FACE_OUTER_BOUND ( 'NONE', #15422, .T. ) ;
#14587=SURFACE_STYLE_USAGE ( .BOTH. , #7416 ) ;
#14596=AXIS2_PLACEMENT_3D ( 'NONE', #7139, #7245, #21253 ) ;
#14603=CARTESIAN_POINT ( 'NONE',  ( 8.181569977154572015, -11.86479625201664412, 7.340676138759426372 ) ) ;
#14616=CARTESIAN_POINT ( 'NONE',  ( 8.079084010241066593, -2.020344040167372679, 6.665520415301748436 ) ) ;
#14628=CIRCLE ( 'NONE', #11612, 0.4999999999999995559 ) ;
#14631=ORIENTED_EDGE ( 'NONE', *, *, #18861, .T. ) ;
#14657=DIRECTION ( 'NONE',  ( -2.168404344970994323E-16, 1.000000000000000000, -1.577721810442023611E-30 ) ) ;
#14661=DIRECTION ( 'NONE',  ( 1.000000000000000000, 2.168404344971017743E-16, -1.780660105995169760E-30 ) ) ;
#14662=CIRCLE ( 'NONE', #1161, 2.549999999999997158 ) ;
#14663=CARTESIAN_POINT ( 'NONE',  ( 7.713464495932034204, -12.17135227947844811, 8.131426806228688520 ) ) ;
#14664=CARTESIAN_POINT ( 'NONE',  ( 8.697224362267997222, -12.00000000000002842, 6.250000000000019540 ) ) ;
#14680=LINE ( 'NONE', #347, #10003 ) ;
#14688=CARTESIAN_POINT ( 'NONE',  ( 7.332081355611500761, -13.77321347121581319, 7.890992604157081480 ) ) ;
#14689=DIRECTION ( 'NONE',  ( 1.000000000000000000, 6.224605580259554159E-31, -2.887593071917436153E-31 ) ) ;
#14701=VECTOR ( 'NONE', #13141, 1000.000000000000000 ) ;
#14706=CARTESIAN_POINT ( 'NONE',  ( 8.129778652391312477, -12.42126101213639444, 7.405931224841370231 ) ) ;
#14710=DIRECTION ( 'NONE',  ( -1.454462294001240516E-30, -1.000000000000000000, -0.000000000000000000 ) ) ;
#14712=LINE ( 'NONE', #7666, #14009 ) ;
#14716=EDGE_CURVE ( 'NONE', #6633, #195, #13169, .T. ) ;
#14718=CARTESIAN_POINT ( 'NONE',  ( -12.85000000000002807, -12.00000000000002842, 6.250000000000019540 ) ) ;
#14726=CARTESIAN_POINT ( 'NONE',  ( 8.148407558030074327, -0.5601289046717625730, 7.382406087063999145 ) ) ;
#14741=ORIENTED_EDGE ( 'NONE', *, *, #15183, .T. ) ;
#14743=CIRCLE ( 'NONE', #15853, 0.4999999999999995559 ) ;
#14751=DIRECTION ( 'NONE',  ( 1.436408664093593395E-16, -0.5454545454545469685, 0.8381404052084432399 ) ) ;
#14754=FACE_OUTER_BOUND ( 'NONE', #14988, .T. ) ;
#14756=DIRECTION ( 'NONE',  ( 1.454462294001240516E-30, 1.000000000000000000, 0.000000000000000000 ) ) ;
#14771=ORIENTED_EDGE ( 'NONE', *, *, #19029, .F. ) ;
#14780=FACE_OUTER_BOUND ( 'NONE', #3358, .T. ) ;
#14794=VECTOR ( 'NONE', #12787, 1000.000000000000000 ) ;
#14807=DIRECTION ( 'NONE',  ( -2.168404344970994323E-16, 1.000000000000000000, -1.577721810442023611E-30 ) ) ;
#14816=B_SPLINE_CURVE_WITH_KNOTS ( 'NONE', 3,
 ( #9263, #7280, #18548, #12665, #16312, #5738, #22081, #3958, #16528, #12910, #215, #2427, #19966, #21739 ),
 .UNSPECIFIED., .F., .F.,
 ( 4, 2, 2, 2, 2, 2, 4 ),
 ( 0.000000000000000000, 0.0008860460682957648024, 0.001772092136591529605, 0.002215115170739412331, 0.002658138204887295492, 0.003101161239035177784, 0.003544184273183060944 ),
 .UNSPECIFIED. ) ;
#14817=AXIS2_PLACEMENT_3D ( 'NONE', #21621, #12655, #9138 ) ;
#14818=EDGE_CURVE ( 'NONE', #9975, #11731, #5315, .T. ) ;
#14825=EDGE_CURVE ( 'NONE', #5698, #13412, #7983, .T. ) ;
#14833=DIRECTION ( 'NONE',  ( 1.000000000000000000, -2.168404344971005170E-16, 1.203141491611682442E-30 ) ) ;
#14849=CARTESIAN_POINT ( 'NONE',  ( 7.490313984279763915, -0.1442844712671001728, 7.566633644154783234 ) ) ;
#14862=DIRECTION ( 'NONE',  ( 0.000000000000000000, 0.000000000000000000, 1.000000000000000000 ) ) ;
#14882=ORIENTED_EDGE ( 'NONE', *, *, #19209, .T. ) ;
#14885=ORIENTED_EDGE ( 'NONE', *, *, #6698, .F. ) ;
#14886=COLOUR_RGB ( '', 0.72549020, 0.75294118, 0.79215686) ;
#14895=CARTESIAN_POINT ( 'NONE',  ( -8.723547172042716014, -11.98401194435532879, 6.817515300136823164 ) ) ;
#14898=AXIS2_PLACEMENT_3D ( 'NONE', #8040, #9801, #4375 ) ;
#14902=TOROIDAL_SURFACE ( 'NONE', #7751, 3.500000000000000000, 0.5000000000000000000 ) ;
#14914=CIRCLE ( 'NONE', #23202, 5.749999999999992006 ) ;
#14923=CARTESIAN_POINT ( 'NONE',  ( 7.920269128372694922, -13.36773923605932346, 7.713069291591548193 ) ) ;
#14925=CARTESIAN_POINT ( 'NONE',  ( -8.954763739086851970, -1.500000000000001332, 6.678571428571422608 ) ) ;
#14941=ADVANCED_FACE ( 'NONE', ( #15732 ), #5211, .T. ) ;
#14957=DIRECTION ( 'NONE',  ( -9.121204216617949000E-31, -1.000000000000000000, 6.982962677686261977E-15 ) ) ;
#14958=CARTESIAN_POINT ( 'NONE',  ( -10.49999999999999467, -13.50000000000000888, 9.250000000000035527 ) ) ;
#14959=ORIENTED_EDGE ( 'NONE', *, *, #22338, .F. ) ;
#14964=ADVANCED_FACE ( 'NONE', ( #10557 ), #17728, .F. ) ;
#14978=CARTESIAN_POINT ( 'NONE',  ( -7.802869476033446716, -2.356467536663312767, 7.917139222842923374 ) ) ;
#14979=EDGE_CURVE ( 'NONE', #20968, #2644, #3724, .T. ) ;
#14988=EDGE_LOOP ( 'NONE', ( #19027, #20785, #11486, #8424, #1463, #16139 ) ) ;
#14996=EDGE_CURVE ( 'NONE', #7710, #8077, #10920, .T. ) ;
#14997=ORIENTED_EDGE ( 'NONE', *, *, #14996, .F. ) ;
#15002=ORIENTED_EDGE ( 'NONE', *, *, #20614, .F. ) ;
#15008=CARTESIAN_POINT ( 'NONE',  ( -8.697224362267972353, -12.00000000000004619, 6.250000000000038192 ) ) ;
#15009=CARTESIAN_POINT ( 'NONE',  ( -8.954763739086862628, -13.50000000000004086, 6.678571428571458135 ) ) ;
#15020=CARTESIAN_POINT ( 'NONE',  ( 12.84999999999997300, -12.00000000000002842, 5.750000000000018652 ) ) ;
#15022=ORIENTED_EDGE ( 'NONE', *, *, #15156, .F. ) ;
#15025=ADVANCED_FACE ( 'NONE', ( #8801 ), #1951, .F. ) ;
#15027=CARTESIAN_POINT ( 'NONE',  ( 8.502135871254301591, -0.5075717384767749474, 6.995667647939175282 ) ) ;
#15028=CARTESIAN_POINT ( 'NONE',  ( -10.49999999999999467, -14.00000000000000888, 9.250000000000035527 ) ) ;
#15029=EDGE_CURVE ( 'NONE', #9714, #7030, #16956, .T. ) ;
#15032=CARTESIAN_POINT ( 'NONE',  ( -10.49999999999999467, -6.938893903907228378E-15, 6.250000000000005329 ) ) ;
#15033=ADVANCED_FACE ( 'NONE', ( #3502 ), #12904, .T. ) ;
#15035=CARTESIAN_POINT ( 'NONE',  ( 8.204963667274169481, -13.91374178095067649, 7.312308861539038141 ) ) ;
#15066=AXIS2_PLACEMENT_3D ( 'NONE', #19964, #12551, #18208 ) ;
#15072=ORIENTED_EDGE ( 'NONE', *, *, #9948, .F. ) ;
#15081=CARTESIAN_POINT ( 'NONE',  ( -7.499999999999987566, -3.018576030000264421, 8.916666666666682062 ) ) ;
#15083=CARTESIAN_POINT ( 'NONE',  ( 7.523705677365597921, -2.838350495275038909, 8.715168381933271036 ) ) ;
#15091=PLANE ( 'NONE',  #22048 ) ;
#15104=VECTOR ( 'NONE', #21507, 1000.000000000000000 ) ;
#15106=CIRCLE ( 'NONE', #463, 5.749999999999992006 ) ;
#15107=B_SPLINE_CURVE_WITH_KNOTS ( 'NONE', 3,
 ( #8626, #15787, #21103, #22986, #6866, #22754, #1230, #17208, #14040, #11914, #21233, #20989, #11806, #18991, #15443, #12254 ),
 .UNSPECIFIED., .F., .F.,
 ( 4, 2, 2, 2, 2, 2, 2, 4 ),
 ( 0.000000000000000000, 0.0008458391445145495551, 0.001268758716771825742, 0.001691678289029102146, 0.002114597861286379200, 0.002537517433543656688, 0.002960437005800934177, 0.003383356578058211665 ),
 .UNSPECIFIED. ) ;
#15117=CARTESIAN_POINT ( 'NONE',  ( -7.324400034341879362, -11.76702354778241499, 7.601326208249701288 ) ) ;
#15120=CARTESIAN_POINT ( 'NONE',  ( -7.748687480237919090, -13.73110298228156978, 8.040801957829067703 ) ) ;
#15127=DIRECTION ( 'NONE',  ( -1.734723475976809806E-16, -1.000000000000000000, 0.000000000000000000 ) ) ;
#15143=VECTOR ( 'NONE', #9431, 1000.000000000000000 ) ;
#15156=EDGE_CURVE ( 'NONE', #14530, #10470, #6458, .T. ) ;
#15164=AXIS2_PLACEMENT_3D ( 'NONE', #3979, #20337, #4201 ) ;
#15166=EDGE_CURVE ( 'NONE', #10359, #20148, #10937, .T. ) ;
#15169=ORIENTED_EDGE ( 'NONE', *, *, #15556, .T. ) ;
#15179=CARTESIAN_POINT ( 'NONE',  ( 8.697224362267997222, -14.00000000000004974, 6.250000000000033751 ) ) ;
#15183=EDGE_CURVE ( 'NONE', #280, #6091, #9378, .T. ) ;
#15186=DIRECTION ( 'NONE',  ( -1.734723475976813750E-16, -1.000000000000000000, 3.469446951953607484E-15 ) ) ;
#15191=ORIENTED_EDGE ( 'NONE', *, *, #22114, .T. ) ;
#15204=CARTESIAN_POINT ( 'NONE',  ( -7.467942433933805191, -2.153931645084739444, 7.356484134531028118 ) ) ;
#15206=CARTESIAN_POINT ( 'NONE',  ( 7.971461718369192262, -2.232205167193722861, 7.625732677302370810 ) ) ;
#15207=CYLINDRICAL_SURFACE ( 'NONE', #17424, 2.549999999999997158 ) ;
#15220=PRODUCT_DEFINITION ( 'UNKNOWN', '', #11621, #20881 ) ;
#15222=CARTESIAN_POINT ( 'NONE',  ( -7.500000000000034639, -12.60977222864646485, 9.250000000000063949 ) ) ;
#15225=DIRECTION ( 'NONE',  ( -2.887593071917436153E-31, -7.888609052210128564E-31, 1.000000000000000000 ) ) ;
#15230=CARTESIAN_POINT ( 'NONE',  ( -7.835522544085319119, -11.94917567266013236, 6.894286109559293330 ) ) ;
#15231=CARTESIAN_POINT ( 'NONE',  ( -8.148407558030072551, -13.43987109532831248, 7.382406087064029343 ) ) ;
#15238=( NAMED_UNIT ( * ) PLANE_ANGLE_UNIT ( ) SI_UNIT ( $, .RADIAN. ) );
#15245=ORIENTED_EDGE ( 'NONE', *, *, #18700, .F. ) ;
#15252=CIRCLE ( 'NONE', #8500, 2.549999999999997158 ) ;
#15253=FACE_OUTER_BOUND ( 'NONE', #8550, .T. ) ;
#15258=CARTESIAN_POINT ( 'NONE',  ( 12.84999999999999964, -13.50000000000011191, -6.249999999999936051 ) ) ;
#15267=DIRECTION ( 'NONE',  ( -1.000000000000000000, -4.252453317207022018E-31, 5.551115123125818447E-17 ) ) ;
#15291=LINE ( 'NONE', #8011, #6507 ) ;
#15299=AXIS2_PLACEMENT_3D ( 'NONE', #922, #4668, #22324 ) ;
#15311=ORIENTED_EDGE ( 'NONE', *, *, #8806, .T. ) ;
#15314=VERTEX_POINT ( 'NONE', #15467 ) ;
#15338=ORIENTED_EDGE ( 'NONE', *, *, #10827, .F. ) ;
#15340=CIRCLE ( 'NONE', #6339, 5.749999999999992006 ) ;
#15356=CARTESIAN_POINT ( 'NONE',  ( -7.120027569165209513, -11.54977705885991668, 8.099087005775032821 ) ) ;
#15381=CARTESIAN_POINT ( 'NONE',  ( -7.029812747553701335, -0.6228290751909227874, 8.933015330925734077 ) ) ;
#15414=EDGE_CURVE ( 'NONE', #13674, #5698, #3081, .T. ) ;
#15422=EDGE_LOOP ( 'NONE', ( #7122, #10743, #13130, #11367 ) ) ;
#15432=CARTESIAN_POINT ( 'NONE',  ( -7.000000000000006217, -5.999999999999974243, 10.24999999999998224 ) ) ;
#15436=CARTESIAN_POINT ( 'NONE',  ( -7.734741761309916086, -2.069990213851658822, 7.004299047562754232 ) ) ;
#15439=CARTESIAN_POINT ( 'NONE',  ( 7.972478112619701740, -1.636497393431803893, 7.628219499134162085 ) ) ;
#15443=CARTESIAN_POINT ( 'NONE',  ( -8.832214555408096857, -12.50000000000003908, 6.752214322824835691 ) ) ;
#15447=CARTESIAN_POINT ( 'NONE',  ( 10.50000000000000888, -1.500000000000001332, 6.250000000000005329 ) ) ;
#15453=ORIENTED_EDGE ( 'NONE', *, *, #4199, .F. ) ;
#15454=EDGE_LOOP ( 'NONE', ( #16567, #14282, #15750, #11523 ) ) ;
#15456=ORIENTED_EDGE ( 'NONE', *, *, #6805, .T. ) ;
#15458=AXIS2_PLACEMENT_3D ( 'NONE', #16645, #9838, #13488 ) ;
#15462=ORIENTED_EDGE ( 'NONE', *, *, #10671, .T. ) ;
#15463=CARTESIAN_POINT ( 'NONE',  ( 6.999999999999992006, 2.775557561562891351E-14, 12.24999999999996980 ) ) ;
#15467=CARTESIAN_POINT ( 'NONE',  ( 7.499999999999992895, -8.000000000000003553, 11.74999999999999645 ) ) ;
#15481=AXIS2_PLACEMENT_3D ( 'NONE', #9780, #21625, #19499 ) ;
#15488=DIRECTION ( 'NONE',  ( 1.000000000000000000, 2.168404344971017743E-16, -1.780660105995169760E-30 ) ) ;
#15495=CARTESIAN_POINT ( 'NONE',  ( -10.49999999999998224, -13.50000000000003020, 5.750000000000032863 ) ) ;
#15496=CARTESIAN_POINT ( 'NONE',  ( -7.748687480237880898, -0.2688970177183537813, 8.040801957829128099 ) ) ;
#15500=VECTOR ( 'NONE', #5869, 1000.000000000000000 ) ;
#15511=AXIS2_PLACEMENT_3D ( 'NONE', #20425, #13596, #2882 ) ;
#15526=VECTOR ( 'NONE', #17144, 1000.000000000000000 ) ;
#15527=AXIS2_PLACEMENT_3D ( 'NONE', #19355, #10296, #9756 ) ;
#15533=CIRCLE ( 'NONE', #5412, 0.4999999999999995559 ) ;
#15543=AXIS2_PLACEMENT_3D ( 'NONE', #193, #11424, #22135 ) ;
#15552=ADVANCED_FACE ( 'NONE', ( #6481 ), #5725, .T. ) ;
#15555=CARTESIAN_POINT ( 'NONE',  ( -8.216162181246556173, -1.557177370613358702, 7.299847320220810509 ) ) ;
#15556=EDGE_CURVE ( 'NONE', #14484, #20416, #13543, .T. ) ;
#15562=AXIS2_PLACEMENT_3D ( 'NONE', #7783, #7362, #734 ) ;
#15563=ADVANCED_FACE ( 'NONE', ( #9897 ), #6374, .T. ) ;
#15597=( LENGTH_UNIT ( ) NAMED_UNIT ( * ) SI_UNIT ( .MILLI., .METRE. ) );
#15614=CARTESIAN_POINT ( 'NONE',  ( -7.856071383949472242, -0.04768060911160423160, 7.015054140272269478 ) ) ;
#15624=DIRECTION ( 'NONE',  ( 1.454462294001240516E-30, 1.000000000000000000, 0.000000000000000000 ) ) ;
#15630=EDGE_LOOP ( 'NONE', ( #4522, #10254, #14997, #5822 ) ) ;
#15633=LINE ( 'NONE', #6709, #8843 ) ;
#15660=CARTESIAN_POINT ( 'NONE',  ( -7.168696526429558347, -0.3737769141893427793, 8.340670630249109152 ) ) ;
#15669=CIRCLE ( 'NONE', #9303, 4.000000000000000000 ) ;
#15696=CARTESIAN_POINT ( 'NONE',  ( -8.137537312224724317, -0.5625089224579539193, 7.396067884835295203 ) ) ;
#15716=B_SPLINE_CURVE_WITH_KNOTS ( 'NONE', 3,
 ( #5535, #19990, #706, #18111, #1986, #9176, #18577, #14688, #3982, #14581, #9632, #4206, #20236, #3865 ),
 .UNSPECIFIED., .F., .F.,
 ( 4, 2, 2, 2, 2, 2, 4 ),
 ( 0.000000000000000000, 0.001011182963765811091, 0.001516774445648716094, 0.002022365927531621314, 0.002527957409414526100, 0.003033548891297431320, 0.004044731855063247832 ),
 .UNSPECIFIED. ) ;
#15721=CARTESIAN_POINT ( 'NONE',  ( -12.85000000000001386, -1.999999999999998224, -6.249999999999992006 ) ) ;
#15726=ADVANCED_FACE ( 'NONE', ( #12367 ), #21331, .F. ) ;
#15728=AXIS2_PLACEMENT_3D ( 'NONE', #1174, #948, #22465 ) ;
#15730=CARTESIAN_POINT ( 'NONE',  ( 12.84999999999997300, -12.00000000000008704, -2.549999999999958966 ) ) ;
#15732=FACE_OUTER_BOUND ( 'NONE', #19244, .T. ) ;
#15738=DIRECTION ( 'NONE',  ( 0.000000000000000000, -7.888609052210128564E-31, 1.000000000000000000 ) ) ;
#15745=ORIENTED_EDGE ( 'NONE', *, *, #7294, .F. ) ;
#15746=EDGE_LOOP ( 'NONE', ( #1351, #16054, #11817, #15462 ) ) ;
#15750=ORIENTED_EDGE ( 'NONE', *, *, #12975, .F. ) ;
#15758=LINE ( 'NONE', #23075, #21072 ) ;
#15766=EDGE_LOOP ( 'NONE', ( #1937, #11891, #1295, #12984 ) ) ;
#15768=VERTEX_POINT ( 'NONE', #3859 ) ;
#15782=CARTESIAN_POINT ( 'NONE',  ( -12.85000000000001386, -12.00000000000006928, 4.163336342344337027E-14 ) ) ;
#15787=CARTESIAN_POINT ( 'NONE',  ( -7.500000000000005329, -11.56013155386942692, 9.052558787159771470 ) ) ;
#15795=( BOUNDED_SURFACE ( )  B_SPLINE_SURFACE ( 3, 2, ( 
 ( #20404, #11566, #6962 ),
 ( #16852, #15083, #22515 ),
 ( #22280, #10155, #11448 ),
 ( #6404, #17204, #8044 ),
 ( #13573, #6174, #18750 ),
 ( #20756, #10041, #2633 ),
 ( #22627, #6286, #9808 ),
 ( #16961, #15206, #8283 ),
 ( #22398, #4510, #15439 ),
 ( #6516, #13691, #4740 ),
 ( #14121, #14242, #16450 ),
 ( #19770, #10818, #21 ),
 ( #8833, #3541, #21433 ),
 ( #129, #10919, #1762 ) ),
 .UNSPECIFIED., .F., .F., .T. ) 
 B_SPLINE_SURFACE_WITH_KNOTS ( ( 4, 2, 2, 2, 2, 2, 4 ),
 ( 3, 3 ),
 ( 2.168404344971008868E-19, 0.0009656398008937972606, 0.001448459701340695837, 0.001931279601787594304, 0.002414099502234492989, 0.002896919402681391240, 0.003862559203575188175 ),
 ( 0.000000000000000000, 1.000000000000000000 ),
 .UNSPECIFIED. ) 
 GEOMETRIC_REPRESENTATION_ITEM ( )  RATIONAL_B_SPLINE_SURFACE ( (
 ( 1.000000000000000000, 0.7071067811865452413, 1.000000000000000000),
 ( 1.000000000000000000, 0.6907538105666497508, 1.000000000000000000),
 ( 1.000000000000000000, 0.6765417438350778134, 1.000000000000000000),
 ( 1.000000000000000000, 0.6623232117677899655, 1.000000000000000000),
 ( 1.000000000000000000, 0.6588386061806286165, 1.000000000000000000),
 ( 1.000000000000000000, 0.6547992448371706686, 1.000000000000000000),
 ( 1.000000000000000000, 0.6542040191407613170, 1.000000000000000000),
 ( 1.000000000000000000, 0.6557724471763412000, 1.000000000000000000),
 ( 1.000000000000000000, 0.6579729115736956402, 1.000000000000000000),
 ( 1.000000000000000000, 0.6644691908065332164, 1.000000000000000000),
 ( 1.000000000000000000, 0.6687559023949577464, 1.000000000000000000),
 ( 1.000000000000000000, 0.6835702420293556791, 1.000000000000000000),
 ( 1.000000000000000000, 0.6960226107070669466, 1.000000000000000000),
 ( 1.000000000000000000, 0.7071067811865451302, 1.000000000000000000) ) ) 
 REPRESENTATION_ITEM ( '' )  SURFACE ( )  );
#15811=ADVANCED_FACE ( 'NONE', ( #17793 ), #11038, .T. ) ;
#15825=AXIS2_PLACEMENT_3D ( 'NONE', #6315, #20548, #18779 ) ;
#15830=CARTESIAN_POINT ( 'NONE',  ( 7.499999999999978684, -1.390227771353540920, 9.250000000000021316 ) ) ;
#15839=CARTESIAN_POINT ( 'NONE',  ( -7.499999999999978684, -8.000000000000010658, 10.74999999999999645 ) ) ;
#15842=CARTESIAN_POINT ( 'NONE',  ( -12.85000000000001386, -12.00000000000005151, 2.550000000000038902 ) ) ;
#15853=AXIS2_PLACEMENT_3D ( 'NONE', #5597, #21251, #1584 ) ;
#15859=EDGE_CURVE ( 'NONE', #19001, #10962, #3451, .T. ) ;
#15870=DIRECTION ( 'NONE',  ( -1.000000000000000000, -4.252453317207022018E-31, 5.551115123125818447E-17 ) ) ;
#15873=TOROIDAL_SURFACE ( 'NONE', #18511, 5.500000000000000000, 0.5000000000000000000 ) ;
#15882=ORIENTED_EDGE ( 'NONE', *, *, #353, .F. ) ;
#15900=CARTESIAN_POINT ( 'NONE',  ( -12.84999999999999964, -13.50000000000003020, 5.750000000000032863 ) ) ;
#15905=CARTESIAN_POINT ( 'NONE',  ( -12.84999999999999964, -12.50000000000011191, -5.749999999999936051 ) ) ;
#15908=AXIS2_PLACEMENT_3D ( 'NONE', #219, #14551, #2080 ) ;
#15910=ORIENTED_EDGE ( 'NONE', *, *, #14109, .F. ) ;
#15912=VECTOR ( 'NONE', #14657, 1000.000000000000000 ) ;
#15915=ORIENTED_EDGE ( 'NONE', *, *, #12972, .T. ) ;
#15934=DIRECTION ( 'NONE',  ( 1.454462294001240516E-30, 1.000000000000000000, 0.000000000000000000 ) ) ;
#15948=EDGE_CURVE ( 'NONE', #6218, #20629, #11271, .T. ) ;
#15951=CARTESIAN_POINT ( 'NONE',  ( 12.84999999999995879, 0.000000000000000000, 5.749999999999991118 ) ) ;
#15956=DIRECTION ( 'NONE',  ( 1.454462294001240516E-30, 1.000000000000000000, 0.000000000000000000 ) ) ;
#15957=PLANE ( 'NONE',  #16724 ) ;
#15965=CARTESIAN_POINT ( 'NONE',  ( -7.499999999999992895, -6.999999999999995559, 11.74999999999999645 ) ) ;
#15968=EDGE_LOOP ( 'NONE', ( #13420, #112, #21588, #17657, #16322, #10089, #422, #10392 ) ) ;
#16000=ORIENTED_EDGE ( 'NONE', *, *, #17720, .T. ) ;
#16011=DIRECTION ( 'NONE',  ( -2.753132232808522832E-17, 0.6666666666666728469, 0.7453559924999245689 ) ) ;
#16013=CARTESIAN_POINT ( 'NONE',  ( 7.644579933246805403, -13.15747815713138991, 8.321099285265846746 ) ) ;
#16016=DIRECTION ( 'NONE',  ( 4.313844246609350428E-33, 6.982962677686276966E-15, 1.000000000000000000 ) ) ;
#16022=CIRCLE ( 'NONE', #18666, 0.4999999999999999445 ) ;
#16025=ORIENTED_EDGE ( 'NONE', *, *, #7180, .F. ) ;
#16032=AXIS2_PLACEMENT_3D ( 'NONE', #14958, #22139, #6030 ) ;
#16053=DIRECTION ( 'NONE',  ( 0.000000000000000000, 0.8381404052084411305, -0.5454545454545505212 ) ) ;
#16054=ORIENTED_EDGE ( 'NONE', *, *, #4199, .T. ) ;
#16058=CIRCLE ( 'NONE', #4042, 2.999999999999995559 ) ;
#16065=CARTESIAN_POINT ( 'NONE',  ( 7.607945571813329089, -0.8975439866889015628, 8.443122311927325541 ) ) ;
#16068=DIRECTION ( 'NONE',  ( 1.000000000000000000, 2.168404344971017743E-16, -1.780660105995169760E-30 ) ) ;
#16071=DIRECTION ( 'NONE',  ( 1.000000000000000000, -2.168404344971017743E-16, 1.203141491611691375E-30 ) ) ;
#16073=CYLINDRICAL_SURFACE ( 'NONE', #20717, 0.4999999999999987232 ) ;
#16083=ORIENTED_EDGE ( 'NONE', *, *, #15029, .T. ) ;
#16089=CIRCLE ( 'NONE', #14596, 5.500000000000000000 ) ;
#16090=EDGE_CURVE ( 'NONE', #396, #16375, #22566, .T. ) ;
#16108=ORIENTED_EDGE ( 'NONE', *, *, #21414, .F. ) ;
#16124=ADVANCED_FACE ( 'NONE', ( #4900 ), #12310, .T. ) ;
#16131=DIRECTION ( 'NONE',  ( 1.454462294001240516E-30, 1.000000000000000000, 0.000000000000000000 ) ) ;
#16135=DIRECTION ( 'NONE',  ( 0.000000000000000000, 6.802837160693368935E-15, 1.000000000000000000 ) ) ;
#16138=CARTESIAN_POINT ( 'NONE',  ( 8.697224362267983011, 1.474514954580286030E-14, 6.250000000000023093 ) ) ;
#16139=ORIENTED_EDGE ( 'NONE', *, *, #13570, .T. ) ;
#16155=CARTESIAN_POINT ( 'NONE',  ( -7.786490775660109165, -13.29349257805250595, 7.963863235126091844 ) ) ;
#16157=CARTESIAN_POINT ( 'NONE',  ( 6.999999999999992006, -8.000000000000051514, 6.249999999999977796 ) ) ;
#16161=LINE ( 'NONE', #1713, #6688 ) ;
#16166=ORIENTED_EDGE ( 'NONE', *, *, #14205, .T. ) ;
#16187=CYLINDRICAL_SURFACE ( 'NONE', #17078, 2.549999999999997158 ) ;
#16206=ORIENTED_EDGE ( 'NONE', *, *, #4401, .T. ) ;
#16212=CARTESIAN_POINT ( 'NONE',  ( -7.271441198316233923, -13.72907106061213689, 8.039702399269760491 ) ) ;
#16229=CARTESIAN_POINT ( 'NONE',  ( -12.84999999999999964, -14.00000000000003020, 5.750000000000032863 ) ) ;
#16232=CARTESIAN_POINT ( 'NONE',  ( 8.719386969281462285, -12.50000000861905214, 6.820015264002557309 ) ) ;
#16235=DIRECTION ( 'NONE',  ( 2.891205793294682961E-15, 0.000000000000000000, 1.000000000000000000 ) ) ;
#16243=AXIS2_PLACEMENT_3D ( 'NONE', #13712, #2770, #13481 ) ;
#16248=DIRECTION ( 'NONE',  ( 0.000000000000000000, 0.000000000000000000, 1.000000000000000000 ) ) ;
#16250=CARTESIAN_POINT ( 'NONE',  ( 7.756475484083233951, -0.06559517125032780782, 7.145789564688715956 ) ) ;
#16256=VERTEX_POINT ( 'NONE', #21624 ) ;
#16287=CIRCLE ( 'NONE', #21176, 0.4999999999999999445 ) ;
#16298=EDGE_LOOP ( 'NONE', ( #9099, #16206, #8904, #17065 ) ) ;
#16307=ADVANCED_FACE ( 'NONE', ( #2301, #8066, #4409 ), #5966, .F. ) ;
#16310=DIRECTION ( 'NONE',  ( -2.168404344971017743E-16, -1.000000000000000000, 6.982962677686261977E-15 ) ) ;
#16312=CARTESIAN_POINT ( 'NONE',  ( -7.268749084027565033, -2.258953384213796767, 7.689023314178085045 ) ) ;
#16317=CIRCLE ( 'NONE', #6191, 0.4999999999999995559 ) ;
#16318=DIRECTION ( 'NONE',  ( 0.000000000000000000, 0.000000000000000000, -1.000000000000000000 ) ) ;
#16322=ORIENTED_EDGE ( 'NONE', *, *, #5410, .T. ) ;
#16328=CARTESIAN_POINT ( 'NONE',  ( 7.576750937466559144, -11.88724926130080206, 7.200086239788022091 ) ) ;
#16333=LINE ( 'NONE', #5763, #14048 ) ;
#16338=CARTESIAN_POINT ( 'NONE',  ( 8.496394830447192348, -13.96748264593550992, 6.998792816379823201 ) ) ;
#16342=DIRECTION ( 'NONE',  ( 0.000000000000000000, 0.000000000000000000, 1.000000000000000000 ) ) ;
#16348=ORIENTED_EDGE ( 'NONE', *, *, #7359, .T. ) ;
#16365=TOROIDAL_SURFACE ( 'NONE', #17100, 5.750000000000000000, 0.5000000000000000000 ) ;
#16366=CARTESIAN_POINT ( 'NONE',  ( 8.697224362267983011, -1.999999999999984457, 6.249999999999992006 ) ) ;
#16368=CARTESIAN_POINT ( 'NONE',  ( 7.651206356577009871, -0.8338323182648625931, 8.300907142094329672 ) ) ;
#16375=VERTEX_POINT ( 'NONE', #10410 ) ;
#16385=DIRECTION ( 'NONE',  ( 9.121204216617949000E-31, 1.000000000000000000, -6.982962677686261977E-15 ) ) ;
#16386=AXIS2_PLACEMENT_3D ( 'NONE', #8312, #17351, #15127 ) ;
#16408=CARTESIAN_POINT ( 'NONE',  ( -7.499999999999992895, -8.000000000000044409, 6.250000000000005329 ) ) ;
#16412=AXIS2_PLACEMENT_3D ( 'NONE', #14348, #359, #8947 ) ;
#16418=CARTESIAN_POINT ( 'NONE',  ( -7.613388670473280051, -13.11165441297978695, 8.423574099071748478 ) ) ;
#16422=AXIS2_PLACEMENT_3D ( 'NONE', #21303, #5533, #7747 ) ;
#16424=CIRCLE ( 'NONE', #11178, 0.4999999999999987232 ) ;
#16437=DIRECTION ( 'NONE',  ( -1.000000000000000000, -6.224605580259554159E-31, 2.887593071917436153E-31 ) ) ;
#16439=CARTESIAN_POINT ( 'NONE',  ( 7.862302507584137956, -11.95343515790908562, 6.866983975782649630 ) ) ;
#16446=DIRECTION ( 'NONE',  ( 9.121204216617949000E-31, 1.000000000000000000, -6.982962677686261977E-15 ) ) ;
#16449=CARTESIAN_POINT ( 'NONE',  ( 7.132286784435703630, -13.57635026841701809, 8.470912490188352351 ) ) ;
#16450=CARTESIAN_POINT ( 'NONE',  ( 8.216162181246719598, -1.557177370613327394, 7.299847320220724356 ) ) ;
#16484=CARTESIAN_POINT ( 'NONE',  ( 7.604097569491915287, -0.4107518873690885752, 8.440516644273330371 ) ) ;
#16494=DIRECTION ( 'NONE',  ( -1.445602896647339163E-16, 1.000000000000000000, -5.348730717595155471E-15 ) ) ;
#16518=EDGE_CURVE ( 'NONE', #16375, #2238, #5374, .T. ) ;
#16520=CARTESIAN_POINT ( 'NONE',  ( 7.499999999999992895, -5.999999999999981348, 10.74999999999998224 ) ) ;
#16528=CARTESIAN_POINT ( 'NONE',  ( -7.862302507584080224, -2.046564842090946801, 6.866983975782588345 ) ) ;
#16545=ORIENTED_EDGE ( 'NONE', *, *, #19156, .T. ) ;
#16547=CYLINDRICAL_SURFACE ( 'NONE', #8118, 0.4999999999999995559 ) ;
#16549=EDGE_CURVE ( 'NONE', #11093, #6727, #14743, .T. ) ;
#16552=DIRECTION ( 'NONE',  ( 1.454462294001240516E-30, 1.000000000000000000, 0.000000000000000000 ) ) ;
#16555=CARTESIAN_POINT ( 'NONE',  ( 8.115139842999440134, -13.89206392873120244, 7.423524081916067274 ) ) ;
#16560=CARTESIAN_POINT ( 'NONE',  ( 6.999999999999978684, -10.98142396999974757, 8.916666666666712260 ) ) ;
#16562=LINE ( 'NONE', #4455, #19091 ) ;
#16567=ORIENTED_EDGE ( 'NONE', *, *, #12388, .T. ) ;
#16568=ORIENTED_EDGE ( 'NONE', *, *, #3492, .F. ) ;
#16569=AXIS2_PLACEMENT_3D ( 'NONE', #15028, #13277, #20459 ) ;
#16570=CARTESIAN_POINT ( 'NONE',  ( -8.697224362268011433, -12.00000000000004263, 6.250000000000019540 ) ) ;
#16572=CARTESIAN_POINT ( 'NONE',  ( 8.518530740350094277, -11.95646899714136957, 6.984205661426876155 ) ) ;
#16575=EDGE_CURVE ( 'NONE', #23124, #20629, #476, .T. ) ;
#16576=CARTESIAN_POINT ( 'NONE',  ( -12.84999999999999964, -0.5000000000000038858, 5.750000000000018652 ) ) ;
#16579=DIRECTION ( 'NONE',  ( 0.000000000000000000, 0.000000000000000000, 1.000000000000000000 ) ) ;
#16589=CARTESIAN_POINT ( 'NONE',  ( 6.999999995223857852, -0.7826352830282113926, 9.233045673661260722 ) ) ;
#16593=VERTEX_POINT ( 'NONE', #1708 ) ;
#16622=VERTEX_POINT ( 'NONE', #20289 ) ;
#16630=ORIENTED_EDGE ( 'NONE', *, *, #1636, .F. ) ;
#16645=CARTESIAN_POINT ( 'NONE',  ( -6.999999999999992006, -8.000000000000044409, 6.250000000000019540 ) ) ;
#16648=CARTESIAN_POINT ( 'NONE',  ( -7.670621117724550686, -11.48840066917088798, 8.215271161873666017 ) ) ;
#16651=CARTESIAN_POINT ( 'NONE',  ( -7.651206356577051615, -13.16616768173521557, 8.300907142094247959 ) ) ;
#16662=ORIENTED_EDGE ( 'NONE', *, *, #11974, .F. ) ;
#16666=ORIENTED_EDGE ( 'NONE', *, *, #22928, .T. ) ;
#16667=CARTESIAN_POINT ( 'NONE',  ( -12.84999999999998721, -12.50000000000002842, 5.750000000000060396 ) ) ;
#16674=CARTESIAN_POINT ( 'NONE',  ( 12.84999999999999964, -2.000000000000005329, -5.749999999999991118 ) ) ;
#16676=CARTESIAN_POINT ( 'NONE',  ( 7.029812747553616958, -13.37717092480913372, 8.933015330925693220 ) ) ;
#16724=AXIS2_PLACEMENT_3D ( 'NONE', #23163, #840, #213 ) ;
#16726=DIRECTION ( 'NONE',  ( 1.454462294001240516E-30, 1.000000000000000000, 0.000000000000000000 ) ) ;
#16728=ORIENTED_EDGE ( 'NONE', *, *, #22846, .T. ) ;
#16729=VERTEX_POINT ( 'NONE', #2398 ) ;
#16731=ADVANCED_FACE ( 'NONE', ( #12992 ), #8188, .T. ) ;
#16735=CARTESIAN_POINT ( 'NONE',  ( -7.725871784772690098, -1.814340584915019372, 8.100883686805044448 ) ) ;
#16737=CARTESIAN_POINT ( 'NONE',  ( 10.49999999999999467, -13.50000000000000888, 9.250000000000063949 ) ) ;
#16741=CIRCLE ( 'NONE', #5135, 5.500000000000000000 ) ;
#16760=CARTESIAN_POINT ( 'NONE',  ( -8.719386969281412547, -12.50000000861904859, 6.820015264002559974 ) ) ;
#16763=DIRECTION ( 'NONE',  ( 0.000000000000000000, -6.938893903907237844E-15, -1.000000000000000000 ) ) ;
#16771=ORIENTED_EDGE ( 'NONE', *, *, #14443, .F. ) ;
#16778=CIRCLE ( 'NONE', #17548, 0.4999999999999995559 ) ;
#16790=CARTESIAN_POINT ( 'NONE',  ( -12.85000000000002807, -12.50000000000002842, 6.250000000000061284 ) ) ;
#16803=CARTESIAN_POINT ( 'NONE',  ( 12.84999999999998721, -12.50000000000002842, 6.250000000000074607 ) ) ;
#16828=EDGE_LOOP ( 'NONE', ( #19239, #2669, #7799, #15882 ) ) ;
#16842=CIRCLE ( 'NONE', #12328, 4.500000000000000888 ) ;
#16844=AXIS2_PLACEMENT_3D ( 'NONE', #17235, #1144, #13606 ) ;
#16852=CARTESIAN_POINT ( 'NONE',  ( 6.999999991928306464, -2.825498329575450551, 8.700799235122079978 ) ) ;
#16862=ADVANCED_FACE ( 'NONE', ( #6854 ), #16993, .T. ) ;
#16881=EDGE_CURVE ( 'NONE', #16729, #13819, #17718, .T. ) ;
#16882=CARTESIAN_POINT ( 'NONE',  ( -7.523705677351674836, -11.16164950472499484, 8.715168381931317043 ) ) ;
#16883=CARTESIAN_POINT ( 'NONE',  ( -8.725359747074561412, -13.50000000719894011, 6.816426071237537521 ) ) ;
#16884=DIRECTION ( 'NONE',  ( -5.551115123125818447E-17, 1.577721810442025713E-30, -1.000000000000000000 ) ) ;
#16901=CARTESIAN_POINT ( 'NONE',  ( 12.84999999999997300, -13.50000000000007105, 5.551115123125782702E-14 ) ) ;
#16921=ORIENTED_EDGE ( 'NONE', *, *, #14996, .T. ) ;
#16937=LINE ( 'NONE', #20732, #19416 ) ;
#16950=CARTESIAN_POINT ( 'NONE',  ( 6.999999999999992006, 2.428612866367529932E-14, 11.74999999999996803 ) ) ;
#16956=B_SPLINE_CURVE_WITH_KNOTS ( 'NONE', 3,
 ( #10675, #1843, #21846, #14545, #21737, #6777, #5623, #17976, #12782, #11131, #14663, #5736, #9031, #20086, #19615, #5395 ),
 .UNSPECIFIED., .F., .F.,
 ( 4, 2, 2, 2, 2, 2, 2, 4 ),
 ( 0.000000000000000000, 0.0004262889904590547608, 0.0008525779809181095216, 0.001278866971377164282, 0.001705155961836219043, 0.002131444952295272720, 0.002557733942754325963, 0.003410311923672432882 ),
 .UNSPECIFIED. ) ;
#16961=CARTESIAN_POINT ( 'NONE',  ( 7.467942433933822066, -2.153931645084771862, 7.356484134531140029 ) ) ;
#16981=EDGE_CURVE ( 'NONE', #10367, #11755, #19273, .T. ) ;
#16990=CARTESIAN_POINT ( 'NONE',  ( -8.954763739086832430, -12.50000000000004263, 6.678571428571468793 ) ) ;
#16991=DIRECTION ( 'NONE',  ( 0.000000000000000000, 0.000000000000000000, -1.000000000000000000 ) ) ;
#16993=TOROIDAL_SURFACE ( 'NONE', #10628, 5.750000000000000000, 0.5000000000000000000 ) ;
#16995=CIRCLE ( 'NONE', #16243, 2.549999999999997158 ) ;
#17016=CARTESIAN_POINT ( 'NONE',  ( -7.500000000000020428, -8.000000000000017764, 10.24999999999999467 ) ) ;
#17025=DIRECTION ( 'NONE',  ( 1.454462294001240516E-30, 1.000000000000000000, 0.000000000000000000 ) ) ;
#17026=CARTESIAN_POINT ( 'NONE',  ( -12.85000000000001386, -12.00000000000006928, 4.163336342344337027E-14 ) ) ;
#17059=CARTESIAN_POINT ( 'NONE',  ( 10.50000000000000888, -13.50000000000003020, 6.250000000000033751 ) ) ;
#17065=ORIENTED_EDGE ( 'NONE', *, *, #19285, .T. ) ;
#17066=ORIENTED_EDGE ( 'NONE', *, *, #8442, .T. ) ;
#17077=CARTESIAN_POINT ( 'NONE',  ( -7.901093513163678139, -1.673173099260699903, 7.745538272134616875 ) ) ;
#17078=AXIS2_PLACEMENT_3D ( 'NONE', #19505, #10788, #19381 ) ;
#17084=LINE ( 'NONE', #10157, #11334 ) ;
#17085=EDGE_CURVE ( 'NONE', #16256, #1201, #2013, .T. ) ;
#17087=DIRECTION ( 'NONE',  ( 0.000000000000000000, 3.469446951953622866E-15, 1.000000000000000000 ) ) ;
#17100=AXIS2_PLACEMENT_3D ( 'NONE', #23216, #7104, #12834 ) ;
#17101=DIRECTION ( 'NONE',  ( 1.454462294001240516E-30, 1.000000000000000000, 0.000000000000000000 ) ) ;
#17112=EDGE_CURVE ( 'NONE', #9040, #15314, #14712, .T. ) ;
#17120=CARTESIAN_POINT ( 'NONE',  ( 10.49999999999998224, -12.00000000000000711, 9.250000000000021316 ) ) ;
#17135=EDGE_CURVE ( 'NONE', #8641, #9717, #15291, .T. ) ;
#17144=DIRECTION ( 'NONE',  ( 1.454462294001240516E-30, 1.000000000000000000, 0.000000000000000000 ) ) ;
#17145=CIRCLE ( 'NONE', #11520, 0.4999999999999995559 ) ;
#17168=DIRECTION ( 'NONE',  ( 1.000000000000000000, 6.224605580259554159E-31, -2.887593071917436153E-31 ) ) ;
#17183=TOROIDAL_SURFACE ( 'NONE', #19441, 5.750000000000000000, 0.5000000000000000000 ) ;
#17190=VECTOR ( 'NONE', #6347, 1000.000000000000000 ) ;
#17203=AXIS2_PLACEMENT_3D ( 'NONE', #21199, #14123, #16342 ) ;
#17204=CARTESIAN_POINT ( 'NONE',  ( 7.670621117724478744, -2.511599330829040966, 8.215271161873941352 ) ) ;
#17208=CARTESIAN_POINT ( 'NONE',  ( -7.884991313526915846, -12.31730826388680455, 7.773664271103684520 ) ) ;
#17235=CARTESIAN_POINT ( 'NONE',  ( -12.85000000000001386, -14.00000000000007105, 5.551115123125782702E-14 ) ) ;
#17241=DIRECTION ( 'NONE',  ( 0.000000000000000000, -6.938893903907237844E-15, -1.000000000000000000 ) ) ;
#17244=EDGE_LOOP ( 'NONE', ( #8060, #15191, #7339, #8530 ) ) ;
#17245=ORIENTED_EDGE ( 'NONE', *, *, #2958, .T. ) ;
#17251=DIRECTION ( 'NONE',  ( -9.121204216617949000E-31, -1.000000000000000000, 6.982962677686261977E-15 ) ) ;
#17276=DIRECTION ( 'NONE',  ( -1.000000000000000000, -2.168404344971017743E-16, 1.780660105995169760E-30 ) ) ;
#17283=CARTESIAN_POINT ( 'NONE',  ( -12.84999999999999964, -1.500000000000001332, 5.750000000000005329 ) ) ;
#17284=EDGE_CURVE ( 'NONE', #17687, #19001, #19975, .T. ) ;
#17307=FACE_OUTER_BOUND ( 'NONE', #15454, .T. ) ;
#17309=DIRECTION ( 'NONE',  ( 1.454462294001240516E-30, 1.000000000000000000, 0.000000000000000000 ) ) ;
#17320=VECTOR ( 'NONE', #3834, 1000.000000000000000 ) ;
#17329=ORIENTED_EDGE ( 'NONE', *, *, #1601, .F. ) ;
#17344=DIRECTION ( 'NONE',  ( -9.121204216617949000E-31, -1.000000000000000000, 6.982962677686261977E-15 ) ) ;
#17350=DIRECTION ( 'NONE',  ( 1.000000000000000000, -2.168404344971005170E-16, 1.203141491611682442E-30 ) ) ;
#17351=DIRECTION ( 'NONE',  ( -1.000000000000000000, 1.734723475976809806E-16, 5.551115123125699502E-17 ) ) ;
#17366=DIRECTION ( 'NONE',  ( 5.551115123125790098E-17, 6.982962677686276177E-15, 1.000000000000000000 ) ) ;
#17369=LINE ( 'NONE', #1282, #20006 ) ;
#17372=CARTESIAN_POINT ( 'NONE',  ( -7.345446946324412529, -0.2181520686730616942, 7.860330092053889217 ) ) ;
#17388=AXIS2_PLACEMENT_3D ( 'NONE', #15782, #3099, #16016 ) ;
#17392=VERTEX_POINT ( 'NONE', #127 ) ;
#17394=CARTESIAN_POINT ( 'NONE',  ( -6.999999999999992006, -8.000000000000044409, 6.250000000000019540 ) ) ;
#17403=CIRCLE ( 'NONE', #15908, 3.499999999999995115 ) ;
#17410=VECTOR ( 'NONE', #17753, 1000.000000000000000 ) ;
#17424=AXIS2_PLACEMENT_3D ( 'NONE', #765, #18751, #7584 ) ;
#17428=CARTESIAN_POINT ( 'NONE',  ( -12.84999999999999964, 0.000000000000000000, 0.000000000000000000 ) ) ;
#17429=DIRECTION ( 'NONE',  ( 0.000000000000000000, -6.938893903907245733E-15, -1.000000000000000000 ) ) ;
#17438=FACE_OUTER_BOUND ( 'NONE', #11518, .T. ) ;
#17456=ORIENTED_EDGE ( 'NONE', *, *, #19000, .F. ) ;
#17473=EDGE_CURVE ( 'NONE', #19925, #8301, #15716, .T. ) ;
#17476=( NAMED_UNIT ( * ) PLANE_ANGLE_UNIT ( ) SI_UNIT ( $, .RADIAN. ) );
#17480=ORIENTED_EDGE ( 'NONE', *, *, #9374, .T. ) ;
#17483=VERTEX_POINT ( 'NONE', #13049 ) ;
#17490=CARTESIAN_POINT ( 'NONE',  ( -12.84999999999999964, -13.50000000000011191, -5.749999999999949374 ) ) ;
#17495=CARTESIAN_POINT ( 'NONE',  ( -7.604097569491801600, -0.4107518873689900429, 8.440516644273033720 ) ) ;
#17498=TOROIDAL_SURFACE ( 'NONE', #23150, 5.750000000000000000, 0.5000000000000000000 ) ;
#17527=VECTOR ( 'NONE', #6681, 1000.000000000000000 ) ;
#17548=AXIS2_PLACEMENT_3D ( 'NONE', #799, #9617, #9271 ) ;
#17559=CARTESIAN_POINT ( 'NONE',  ( 12.84999999999997300, -12.00000000000006928, 4.163336342344337027E-14 ) ) ;
#17566=EDGE_LOOP ( 'NONE', ( #3578, #16728, #8441, #8446 ) ) ;
#17569=EDGE_LOOP ( 'NONE', ( #12080, #111, #247, #20506, #2622, #13924 ) ) ;
#17582=EDGE_CURVE ( 'NONE', #6218, #5465, #9558, .T. ) ;
#17610=EDGE_CURVE ( 'NONE', #9040, #20589, #7289, .T. ) ;
#17642=ADVANCED_FACE ( 'NONE', ( #11620 ), #18809, .T. ) ;
#17643=CARTESIAN_POINT ( 'NONE',  ( -7.168696526429614302, -13.62622308581068253, 8.340670630249134021 ) ) ;
#17654=ORIENTED_EDGE ( 'NONE', *, *, #14979, .T. ) ;
#17657=ORIENTED_EDGE ( 'NONE', *, *, #5862, .T. ) ;
#17659=DIRECTION ( 'NONE',  ( -1.000000000000000000, -1.910522504832140594E-31, 5.551115123125818447E-17 ) ) ;
#17687=VERTEX_POINT ( 'NONE', #7018 ) ;
#17688=ORIENTED_EDGE ( 'NONE', *, *, #18745, .T. ) ;
#17698=CIRCLE ( 'NONE', #3065, 0.4999999999999987232 ) ;
#17712=ORIENTED_EDGE ( 'NONE', *, *, #22928, .F. ) ;
#17718=B_SPLINE_CURVE_WITH_KNOTS ( 'NONE', 3,
 ( #1443, #8857, #5323, #10606, #16013, #17912, #14030, #43, #3564, #10726, #9077, #8618, #1788, #21569 ),
 .UNSPECIFIED., .F., .F.,
 ( 4, 2, 2, 2, 2, 2, 4 ),
 ( 1.176546704354857500E-17, 0.0008155857435326490431, 0.001223378615298965216, 0.001631171487065281823, 0.002038964358831596695, 0.002446757230597911784, 0.003262342974130545432 ),
 .UNSPECIFIED. ) ;
#17720=EDGE_CURVE ( 'NONE', #11726, #11691, #8774, .T. ) ;
#17726=DIRECTION ( 'NONE',  ( 1.000000000000000000, -2.168404344971005170E-16, 1.203141491611682442E-30 ) ) ;
#17728=CYLINDRICAL_SURFACE ( 'NONE', #9069, 2.999999999999995559 ) ;
#17736=VECTOR ( 'NONE', #10321, 1000.000000000000000 ) ;
#17753=DIRECTION ( 'NONE',  ( 5.551115123125761132E-17, -1.577721810442025713E-30, 1.000000000000000000 ) ) ;
#17761=CARTESIAN_POINT ( 'NONE',  ( -12.85000000000002807, -1.999999999999998224, 6.249999999999950262 ) ) ;
#17762=PLANE ( 'NONE',  #16422 ) ;
#17775=AXIS2_PLACEMENT_3D ( 'NONE', #1468, #13930, #10288 ) ;
#17776=ADVANCED_FACE ( 'NONE', ( #413 ), #15207, .F. ) ;
#17791=CARTESIAN_POINT ( 'NONE',  ( -6.999999999999992006, -12.60977222864646485, 9.250000000000078160 ) ) ;
#17793=FACE_OUTER_BOUND ( 'NONE', #7062, .T. ) ;
#17798=AXIS2_PLACEMENT_3D ( 'NONE', #16737, #2983, #22279 ) ;
#17811=VECTOR ( 'NONE', #22783, 1000.000000000000000 ) ;
#17813=AXIS2_PLACEMENT_3D ( 'NONE', #18036, #16131, #8979 ) ;
#17818=ORIENTED_EDGE ( 'NONE', *, *, #6535, .F. ) ;
#17825=CARTESIAN_POINT ( 'NONE',  ( 7.499999999999978684, -1.390227771353540920, 9.250000000000021316 ) ) ;
#17827=DIRECTION ( 'NONE',  ( -2.753132232808505576E-17, 0.6666666666666667407, -0.7453559924999297870 ) ) ;
#17828=EDGE_CURVE ( 'NONE', #5440, #15768, #4511, .T. ) ;
#17830=DIRECTION ( 'NONE',  ( 1.000000000000000000, 1.910522504832140594E-31, -5.551115123125818447E-17 ) ) ;
#17831=AXIS2_PLACEMENT_3D ( 'NONE', #1657, #5066, #12222 ) ;
#17851=CARTESIAN_POINT ( 'NONE',  ( 12.84999999999997300, -14.00000000000003020, 5.750000000000032863 ) ) ;
#17859=FACE_OUTER_BOUND ( 'NONE', #2530, .T. ) ;
#17908=CARTESIAN_POINT ( 'NONE',  ( 7.638377885296781855, -12.06377841978598831, 8.340398698103349773 ) ) ;
#17909=CARTESIAN_POINT ( 'NONE',  ( -8.438463404362684273, -11.99816466695113526, 6.398712851742201835 ) ) ;
#17912=CARTESIAN_POINT ( 'NONE',  ( 7.733764002503177970, -13.25269934883866441, 8.082002268151514457 ) ) ;
#17918=CYLINDRICAL_SURFACE ( 'NONE', #23013, 0.4999999999999995559 ) ;
#17922=CARTESIAN_POINT ( 'NONE',  ( 7.026577802269673434, -2.648906230146660601, 8.453373545151620760 ) ) ;
#17924=CARTESIAN_POINT ( 'NONE',  ( 7.525553787417718965, -1.070926652787001609, 8.786654903594095956 ) ) ;
#17930=ORIENTED_EDGE ( 'NONE', *, *, #11252, .T. ) ;
#17931=EDGE_LOOP ( 'NONE', ( #17245, #9021, #13902, #5750 ) ) ;
#17934=ORIENTED_EDGE ( 'NONE', *, *, #11241, .T. ) ;
#17955=CIRCLE ( 'NONE', #7420, 0.4999999999999995559 ) ;
#17969=CARTESIAN_POINT ( 'NONE',  ( 7.644579933246795633, -0.8425218428686449545, 8.321099285265821877 ) ) ;
#17976=CARTESIAN_POINT ( 'NONE',  ( 7.955953741309954808, -12.35582749618195741, 7.654083333123934629 ) ) ;
#17978=CARTESIAN_POINT ( 'NONE',  ( 10.49999999999998224, -0.5000000000000004441, 6.250000000000061284 ) ) ;
#17998=CIRCLE ( 'NONE', #18722, 0.5000000000000002220 ) ;
#18022=ORIENTED_EDGE ( 'NONE', *, *, #9374, .F. ) ;
#18029=CARTESIAN_POINT ( 'NONE',  ( -7.761744141695584354, -11.93564195219169477, 6.973942750959578163 ) ) ;
#18036=CARTESIAN_POINT ( 'NONE',  ( -12.84999999999999964, -2.000000000000001776, 0.000000000000000000 ) ) ;
#18045=CARTESIAN_POINT ( 'NONE',  ( 7.490952241692643732, -0.6544882962155422756, 8.992386117842515958 ) ) ;
#18046=EDGE_LOOP ( 'NONE', ( #540, #5531, #14537, #20040 ) ) ;
#18058=ORIENTED_EDGE ( 'NONE', *, *, #4501, .F. ) ;
#18060=CARTESIAN_POINT ( 'NONE',  ( -10.49999999999998224, -12.50000000000002842, 6.250000000000061284 ) ) ;
#18069=AXIS2_PLACEMENT_3D ( 'NONE', #1081, #13657, #9773 ) ;
#18073=CARTESIAN_POINT ( 'NONE',  ( -10.49999999999999467, -13.50000000000000888, 9.250000000000035527 ) ) ;
#18079=EDGE_CURVE ( 'NONE', #19457, #3351, #12917, .T. ) ;
#18099=LINE ( 'NONE', #18332, #10243 ) ;
#18111=CARTESIAN_POINT ( 'NONE',  ( 7.835312244870012321, -13.94896639302768371, 7.041165740960589225 ) ) ;
#18112=EDGE_CURVE ( 'NONE', #6039, #21059, #2777, .T. ) ;
#18123=VERTEX_POINT ( 'NONE', #47 ) ;
#18137=FACE_OUTER_BOUND ( 'NONE', #22300, .T. ) ;
#18138=DIRECTION ( 'NONE',  ( -1.454462294001240516E-30, -1.000000000000000000, -0.000000000000000000 ) ) ;
#18147=AXIS2_PLACEMENT_3D ( 'NONE', #4870, #12040, #1362 ) ;
#18155=CARTESIAN_POINT ( 'NONE',  ( 7.568268608012000520, -0.4673147976723873165, 8.579161250779968384 ) ) ;
#18172=AXIS2_PLACEMENT_3D ( 'NONE', #19394, #10340, #7177 ) ;
#18175=ADVANCED_FACE ( 'NONE', ( #21906 ), #11073, .T. ) ;
#18182=CARTESIAN_POINT ( 'NONE',  ( 7.000000000000006217, -5.999999999999981348, 6.250000000000005329 ) ) ;
#18201=ORIENTED_EDGE ( 'NONE', *, *, #17085, .T. ) ;
#18203=AXIS2_PLACEMENT_3D ( 'NONE', #14498, #23223, #9204 ) ;
#18208=DIRECTION ( 'NONE',  ( 0.000000000000000000, 0.000000000000000000, -1.000000000000000000 ) ) ;
#18223=EDGE_LOOP ( 'NONE', ( #14428, #8693, #6031, #11216 ) ) ;
#18239=DIRECTION ( 'NONE',  ( -1.000000000000000000, -1.910522504832140594E-31, 5.551115123125818447E-17 ) ) ;
#18241=CIRCLE ( 'NONE', #1342, 2.549999999999997158 ) ;
#18250=CARTESIAN_POINT ( 'NONE',  ( 8.037202331403122457, -11.80340871766173017, 7.528743044528821926 ) ) ;
#18251=CARTESIAN_POINT ( 'NONE',  ( -7.491585531133571507, -11.85620892266377702, 7.320610673787158795 ) ) ;
#18253=DIRECTION ( 'NONE',  ( 0.000000000000000000, 0.000000000000000000, 1.000000000000000000 ) ) ;
#18265=CARTESIAN_POINT ( 'NONE',  ( 7.796097383573778572, -0.6999727310043983852, 7.943830786858195658 ) ) ;
#18274=ORIENTED_EDGE ( 'NONE', *, *, #14291, .T. ) ;
#18280=VECTOR ( 'NONE', #5992, 1000.000000000000000 ) ;
#18317=CIRCLE ( 'NONE', #4396, 3.499999999999995115 ) ;
#18320=CARTESIAN_POINT ( 'NONE',  ( 7.884991313526934498, -1.682691736113213432, 7.773664271103622347 ) ) ;
#18322=DIRECTION ( 'NONE',  ( 1.000000000000000000, 4.252453317207022018E-31, -5.551115123125818447E-17 ) ) ;
#18328=VERTEX_POINT ( 'NONE', #8253 ) ;
#18332=CARTESIAN_POINT ( 'NONE',  ( 10.50000000000000888, -1.999999999999984457, 6.250000000000005329 ) ) ;
#18338=CARTESIAN_POINT ( 'NONE',  ( 8.954763739086823549, -0.5000000000000004441, 6.678571428571450141 ) ) ;
#18344=CARTESIAN_POINT ( 'NONE',  ( -10.49999999999996803, -0.5000000000000004441, 9.250000000000035527 ) ) ;
#18347=CARTESIAN_POINT ( 'NONE',  ( -10.49999999999998224, -0.5000000000000038858, 5.750000000000032863 ) ) ;
#18352=SURFACE_STYLE_FILL_AREA ( #3988 ) ;
#18363=EDGE_LOOP ( 'NONE', ( #2276, #20411, #8002, #16348 ) ) ;
#18369=CARTESIAN_POINT ( 'NONE',  ( 8.422565759993609902, -12.00000000000004796, 6.396710472006761350 ) ) ;
#18382=CARTESIAN_POINT ( 'NONE',  ( 6.999999999999978684, -3.018576030000261312, 8.916666666666724694 ) ) ;
#18384=CARTESIAN_POINT ( 'NONE',  ( 7.694134585029391182, -0.3119908745745466616, 8.172315317060892426 ) ) ;
#18388=ORIENTED_EDGE ( 'NONE', *, *, #12245, .T. ) ;
#18389=ORIENTED_EDGE ( 'NONE', *, *, #18965, .T. ) ;
#18400=CARTESIAN_POINT ( 'NONE',  ( -7.602880770961763623, -2.006500808705121486, 8.461619612152039949 ) ) ;
#18410=ADVANCED_FACE ( 'NONE', ( #10015 ), #21601, .T. ) ;
#18412=ORIENTED_EDGE ( 'NONE', *, *, #12002, .T. ) ;
#18428=CARTESIAN_POINT ( 'NONE',  ( -8.260108127873365902, -11.89083139210929296, 7.249251683976637217 ) ) ;
#18430=CARTESIAN_POINT ( 'NONE',  ( -7.525553787417716300, -12.92907334721332013, 8.786654903594138588 ) ) ;
#18471=AXIS2_PLACEMENT_3D ( 'NONE', #5320, #12239, #5207 ) ;
#18476=FACE_OUTER_BOUND ( 'NONE', #56, .T. ) ;
#18477=LINE ( 'NONE', #2360, #6429 ) ;
#18487=LINE ( 'NONE', #5909, #1056 ) ;
#18492=EDGE_CURVE ( 'NONE', #9721, #9717, #19713, .T. ) ;
#18495=ORIENTED_EDGE ( 'NONE', *, *, #12335, .T. ) ;
#18511=AXIS2_PLACEMENT_3D ( 'NONE', #16157, #6652, #12402 ) ;
#18544=AXIS2_PLACEMENT_3D ( 'NONE', #17761, #8942, #19765 ) ;
#18546=CARTESIAN_POINT ( 'NONE',  ( -8.216162181246543739, -12.44282262938666328, 7.299847320220930413 ) ) ;
#18547=VECTOR ( 'NONE', #10122, 1000.000000000000000 ) ;
#18548=CARTESIAN_POINT ( 'NONE',  ( -7.026577802269633466, -2.648906230146649943, 8.453373545151602997 ) ) ;
#18577=CARTESIAN_POINT ( 'NONE',  ( 7.473326079327807570, -13.84852298796451997, 7.598194856234284700 ) ) ;
#18578=CARTESIAN_POINT ( 'NONE',  ( 7.991520206789753722, -13.39565235458638881, 7.599114430427904132 ) ) ;
#18596=CARTESIAN_POINT ( 'NONE',  ( -6.999999999999992006, -5.999999999999987566, 6.250000000000005329 ) ) ;
#18606=DIRECTION ( 'NONE',  ( 6.656013887802287108E-31, 1.000000000000000000, -3.469446951953609061E-15 ) ) ;
#18617=ORIENTED_EDGE ( 'NONE', *, *, #5410, .F. ) ;
#18633=CARTESIAN_POINT ( 'NONE',  ( -7.499999999999992895, -5.999999999999987566, 6.249999999999992006 ) ) ;
#18635=CARTESIAN_POINT ( 'NONE',  ( -7.000000000000006217, -6.999999999999995559, 10.75000000000000888 ) ) ;
#18641=VERTEX_POINT ( 'NONE', #16560 ) ;
#18648=EDGE_LOOP ( 'NONE', ( #14429, #9101, #11544, #1531 ) ) ;
#18657=CARTESIAN_POINT ( 'NONE',  ( -8.954763739086862628, -14.00000000000004441, 6.678571428571461688 ) ) ;
#18666=AXIS2_PLACEMENT_3D ( 'NONE', #1344, #19560, #19687 ) ;
#18671=ORIENTED_EDGE ( 'NONE', *, *, #4454, .T. ) ;
#18693=CIRCLE ( 'NONE', #6314, 0.4999999999999995559 ) ;
#18699=APPLICATION_CONTEXT ( 'automotive_design' ) ;
#18700=EDGE_CURVE ( 'NONE', #22681, #14484, #6460, .T. ) ;
#18704=LINE ( 'NONE', #11875, #18547 ) ;
#18708=CARTESIAN_POINT ( 'NONE',  ( 6.999999999999992006, -8.000000000000051514, 6.249999999999977796 ) ) ;
#18720=CIRCLE ( 'NONE', #17203, 3.499999999999996003 ) ;
#18722=AXIS2_PLACEMENT_3D ( 'NONE', #11101, #14751, #7814 ) ;
#18745=EDGE_CURVE ( 'NONE', #20539, #20452, #8336, .T. ) ;
#18750=CARTESIAN_POINT ( 'NONE',  ( 7.638377885296685932, -1.936221580214098292, 8.340398698103570041 ) ) ;
#18751=DIRECTION ( 'NONE',  ( 1.454462294001240516E-30, 1.000000000000000000, 0.000000000000000000 ) ) ;
#18758=FACE_OUTER_BOUND ( 'NONE', #10972, .T. ) ;
#18759=EDGE_LOOP ( 'NONE', ( #15072, #2851 ) ) ;
#18763=TOROIDAL_SURFACE ( 'NONE', #2597, 4.500000000000000888, 0.5000000000000000000 ) ;
#18767=ORIENTED_EDGE ( 'NONE', *, *, #4501, .T. ) ;
#18779=DIRECTION ( 'NONE',  ( 0.000000000000000000, 0.000000000000000000, 1.000000000000000000 ) ) ;
#18787=SURFACE_SIDE_STYLE ('',( #8080 ) ) ;
#18809=CYLINDRICAL_SURFACE ( 'NONE', #3157, 6.249999999999992006 ) ;
#18813=CARTESIAN_POINT ( 'NONE',  ( -12.84999999999999964, -0.5000000000000038858, 6.250000000000033751 ) ) ;
#18822=DIRECTION ( 'NONE',  ( 0.000000000000000000, 6.802837160693368935E-15, 1.000000000000000000 ) ) ;
#18832=DIRECTION ( 'NONE',  ( 1.000000000000000000, -2.168404344971005170E-16, 1.203141491611682442E-30 ) ) ;
#18836=DIRECTION ( 'NONE',  ( 2.891205793294678326E-16, 1.000000000000000000, 0.000000000000000000 ) ) ;
#18857=DIRECTION ( 'NONE',  ( 0.5150787536377134934, 0.000000000000000000, -0.8571428571428567622 ) ) ;
#18861=EDGE_CURVE ( 'NONE', #5698, #20776, #5773, .T. ) ;
#18870=PRODUCT ( 'Link', 'Link', '', ( #11055 ) ) ;
#18881=AXIS2_PLACEMENT_3D ( 'NONE', #10870, #16385, #14296 ) ;
#18884=CIRCLE ( 'NONE', #21144, 5.749999999999992006 ) ;
#18887=CARTESIAN_POINT ( 'NONE',  ( 10.50000000000000888, -2.000000000000001776, 5.750000000000005329 ) ) ;
#18897=CARTESIAN_POINT ( 'NONE',  ( -7.161440864725725497, -11.61224748569070364, 7.973376427817314038 ) ) ;
#18902=DIRECTION ( 'NONE',  ( 1.000000000000000000, 2.168404344971017743E-16, -1.780660105995169760E-30 ) ) ;
#18908=SURFACE_STYLE_USAGE ( .BOTH. , #18787 ) ;
#18911=VERTEX_POINT ( 'NONE', #15842 ) ;
#18924=DIRECTION ( 'NONE',  ( 2.168404344970994323E-16, -1.000000000000000000, 1.577721810442023611E-30 ) ) ;
#18942=VERTEX_POINT ( 'NONE', #10330 ) ;
#18965=EDGE_CURVE ( 'NONE', #17392, #21322, #809, .T. ) ;
#18977=DIRECTION ( 'NONE',  ( 0.000000000000000000, 3.469446951953616555E-15, 1.000000000000000000 ) ) ;
#18989=CARTESIAN_POINT ( 'NONE',  ( -7.000000000000020428, -8.000000000000010658, 10.74999999999998224 ) ) ;
#18991=CARTESIAN_POINT ( 'NONE',  ( -8.715898959466873208, -12.49756837761075978, 6.833978265954060660 ) ) ;
#18994=ORIENTED_EDGE ( 'NONE', *, *, #22390, .F. ) ;
#19000=EDGE_CURVE ( 'NONE', #12774, #21109, #2430, .T. ) ;
#19001=VERTEX_POINT ( 'NONE', #10898 ) ;
#19003=EDGE_LOOP ( 'NONE', ( #13903, #12922 ) ) ;
#19007=AXIS2_PLACEMENT_3D ( 'NONE', #153, #16011, #7890 ) ;
#19011=DIRECTION ( 'NONE',  ( -1.000000000000000000, -4.252453317207022018E-31, 5.551115123125818447E-17 ) ) ;
#19027=ORIENTED_EDGE ( 'NONE', *, *, #3989, .T. ) ;
#19028=VECTOR ( 'NONE', #18322, 1000.000000000000000 ) ;
#19029=EDGE_CURVE ( 'NONE', #4343, #19925, #17403, .T. ) ;
#19043=EDGE_CURVE ( 'NONE', #12774, #22329, #7387, .T. ) ;
#19049=LINE ( 'NONE', #21282, #14178 ) ;
#19052=EDGE_CURVE ( 'NONE', #21109, #16622, #2202, .T. ) ;
#19061=ORIENTED_EDGE ( 'NONE', *, *, #18112, .T. ) ;
#19074=EDGE_CURVE ( 'NONE', #4924, #7803, #9915, .T. ) ;
#19081=ORIENTED_EDGE ( 'NONE', *, *, #10671, .F. ) ;
#19090=CARTESIAN_POINT ( 'NONE',  ( -7.972478112619597823, -1.636497393431879610, 7.628219499134209158 ) ) ;
#19091=VECTOR ( 'NONE', #18239, 1000.000000000000000 ) ;
#19095=DIRECTION ( 'NONE',  ( -1.000000000000000000, -6.224605580259554159E-31, 2.887593071917436153E-31 ) ) ;
#19101=DIRECTION ( 'NONE',  ( 1.454462294001240516E-30, 1.000000000000000000, 0.000000000000000000 ) ) ;
#19110=ORIENTED_EDGE ( 'NONE', *, *, #22146, .F. ) ;
#19122=CARTESIAN_POINT ( 'NONE',  ( -8.510464245293324126, -13.49280278100719421, 6.988717072694019095 ) ) ;
#19133=ORIENTED_EDGE ( 'NONE', *, *, #2620, .F. ) ;
#19142=ORIENTED_EDGE ( 'NONE', *, *, #2958, .F. ) ;
#19143=CARTESIAN_POINT ( 'NONE',  ( -12.85000000000001386, -1.499999999999997780, -5.749999999999976907 ) ) ;
#19151=CARTESIAN_POINT ( 'NONE',  ( -7.500000000000020428, -1.390227771353544473, 9.250000000000014211 ) ) ;
#19154=CARTESIAN_POINT ( 'NONE',  ( 7.499999999999978684, -8.000000000000051514, 6.249999999999977796 ) ) ;
#19156=EDGE_CURVE ( 'NONE', #19457, #11731, #13254, .T. ) ;
#19164=VERTEX_POINT ( 'NONE', #22428 ) ;
#19178=CARTESIAN_POINT ( 'NONE',  ( -12.84999999999999964, 0.000000000000000000, 0.000000000000000000 ) ) ;
#19181=EDGE_CURVE ( 'NONE', #20452, #22613, #14434, .T. ) ;
#19186=DIRECTION ( 'NONE',  ( 1.000000000000000000, -2.168404344971005170E-16, 1.203141491611682442E-30 ) ) ;
#19188=ORIENTED_EDGE ( 'NONE', *, *, #617, .F. ) ;
#19199=FACE_OUTER_BOUND ( 'NONE', #20075, .T. ) ;
#19209=EDGE_CURVE ( 'NONE', #8301, #2644, #20446, .T. ) ;
#19226=VECTOR ( 'NONE', #18924, 1000.000000000000000 ) ;
#19229=CARTESIAN_POINT ( 'NONE',  ( -8.718376657154855991, -13.50000000000003553, 6.820622386032004769 ) ) ;
#19239=ORIENTED_EDGE ( 'NONE', *, *, #17135, .F. ) ;
#19244=EDGE_LOOP ( 'NONE', ( #18671, #19312, #20715, #15910 ) ) ;
#19260=CARTESIAN_POINT ( 'NONE',  ( -7.876571740167083391, -0.1939399797844225393, 7.785394814390953044 ) ) ;
#19263=DIRECTION ( 'NONE',  ( 0.000000000000000000, -3.469446951953616555E-15, -1.000000000000000000 ) ) ;
#19273=CIRCLE ( 'NONE', #8754, 6.249999999999992006 ) ;
#19282=ORIENTED_EDGE ( 'NONE', *, *, #9572, .T. ) ;
#19285=EDGE_CURVE ( 'NONE', #9040, #9710, #21491, .T. ) ;
#19299=VECTOR ( 'NONE', #11123, 1000.000000000000000 ) ;
#19312=ORIENTED_EDGE ( 'NONE', *, *, #17582, .F. ) ;
#19323=DIRECTION ( 'NONE',  ( 0.000000000000000000, 0.000000000000000000, 1.000000000000000000 ) ) ;
#19325=CARTESIAN_POINT ( 'NONE',  ( -7.473326079327731186, -0.1514770120355157235, 7.598194856234254502 ) ) ;
#19347=DIRECTION ( 'NONE',  ( 0.000000000000000000, 0.000000000000000000, 1.000000000000000000 ) ) ;
#19355=CARTESIAN_POINT ( 'NONE',  ( 6.999999999999992006, -8.000000000000010658, 10.74999999999999645 ) ) ;
#19379=CARTESIAN_POINT ( 'NONE',  ( -7.525553787417682550, -1.070926652787118405, 8.786654903594046218 ) ) ;
#19381=DIRECTION ( 'NONE',  ( 0.000000000000000000, 6.802837160693368935E-15, 1.000000000000000000 ) ) ;
#19391=DIRECTION ( 'NONE',  ( 0.000000000000000000, 0.000000000000000000, 1.000000000000000000 ) ) ;
#19394=CARTESIAN_POINT ( 'NONE',  ( 12.84999999999997300, 0.000000000000000000, 1.387778780781445676E-14 ) ) ;
#19407=ADVANCED_FACE ( 'NONE', ( #21715 ), #82, .T. ) ;
#19412=EDGE_CURVE ( 'NONE', #7030, #16729, #6027, .T. ) ;
#19416=VECTOR ( 'NONE', #15186, 1000.000000000000000 ) ;
#19419=VERTEX_POINT ( 'NONE', #1931 ) ;
#19431=DIRECTION ( 'NONE',  ( -4.019602852144215652E-47, -6.982962677686261977E-15, -1.000000000000000000 ) ) ;
#19432=VECTOR ( 'NONE', #10795, 1000.000000000000000 ) ;
#19441=AXIS2_PLACEMENT_3D ( 'NONE', #7448, #10852, #16248 ) ;
#19444=ADVANCED_FACE ( 'NONE', ( #618 ), #11536, .T. ) ;
#19457=VERTEX_POINT ( 'NONE', #13196 ) ;
#19459=EDGE_LOOP ( 'NONE', ( #17712, #23180 ) ) ;
#19491=ORIENTED_EDGE ( 'NONE', *, *, #877, .F. ) ;
#19495=CARTESIAN_POINT ( 'NONE',  ( 8.137537312224758068, -0.5625089224579603586, 7.396067884835346717 ) ) ;
#19499=DIRECTION ( 'NONE',  ( 0.000000000000000000, 0.000000000000000000, 1.000000000000000000 ) ) ;
#19500=CARTESIAN_POINT ( 'NONE',  ( 12.84999999999997300, -12.00000000000006928, 4.163336342344337027E-14 ) ) ;
#19502=CARTESIAN_POINT ( 'NONE',  ( -8.697224362267961695, 1.160096324559489744E-14, 6.249999999999961808 ) ) ;
#19505=CARTESIAN_POINT ( 'NONE',  ( 12.84999999999997300, -12.00000000000006928, 4.163336342344337027E-14 ) ) ;
#19513=DIRECTION ( 'NONE',  ( -1.000000000000000000, -6.224605580259554159E-31, 2.887593071917436153E-31 ) ) ;
#19516=VERTEX_POINT ( 'NONE', #1113 ) ;
#19532=CARTESIAN_POINT ( 'NONE',  ( -12.85000000000001386, 0.000000000000000000, -5.749999999999991118 ) ) ;
#19535=CARTESIAN_POINT ( 'NONE',  ( -12.84999999999999964, -13.50000000000003020, 5.750000000000032863 ) ) ;
#19541=ORIENTED_EDGE ( 'NONE', *, *, #7294, .T. ) ;
#19552=CARTESIAN_POINT ( 'NONE',  ( -7.126417736726627261, -0.4330224014298838520, 8.494066294656311911 ) ) ;
#19554=CYLINDRICAL_SURFACE ( 'NONE', #5252, 6.249999999999992006 ) ;
#19555=FACE_OUTER_BOUND ( 'NONE', #4108, .T. ) ;
#19560=DIRECTION ( 'NONE',  ( 0.8571428571428572063, -1.183291357831519285E-30, 0.5150787536377126052 ) ) ;
#19568=ORIENTED_EDGE ( 'NONE', *, *, #16575, .T. ) ;
#19580=FACE_OUTER_BOUND ( 'NONE', #2877, .T. ) ;
#19584=DIRECTION ( 'NONE',  ( 1.000000000000000000, 6.224605580259554159E-31, -2.887593071917436153E-31 ) ) ;
#19587=DIRECTION ( 'NONE',  ( -2.168404344971008868E-16, 1.000000000000000000, 0.000000000000000000 ) ) ;
#19603=AXIS2_PLACEMENT_3D ( 'NONE', #6850, #8730, #20104 ) ;
#19613=DIRECTION ( 'NONE',  ( 0.000000000000000000, -6.938893903907237844E-15, -1.000000000000000000 ) ) ;
#19615=CARTESIAN_POINT ( 'NONE',  ( 7.500000000000007105, -11.56013155386943758, 9.052558787159764364 ) ) ;
#19658=TOROIDAL_SURFACE ( 'NONE', #4617, 5.500000000000000000, 0.5000000000000000000 ) ;
#19661=ORIENTED_EDGE ( 'NONE', *, *, #9543, .F. ) ;
#19663=ADVANCED_FACE ( 'NONE', ( #19555 ), #14452, .T. ) ;
#19670=CARTESIAN_POINT ( 'NONE',  ( 7.024848138041158485, -11.34038014973665476, 8.468562630484207432 ) ) ;
#19680=CIRCLE ( 'NONE', #525, 2.549999999999997158 ) ;
#19681=DIRECTION ( 'NONE',  ( -1.454462294001240516E-30, -1.000000000000000000, -0.000000000000000000 ) ) ;
#19682=CARTESIAN_POINT ( 'NONE',  ( -10.49999999999996803, -1.500000000000001332, 9.250000000000008882 ) ) ;
#19687=DIRECTION ( 'NONE',  ( 0.5150787536377134934, 0.000000000000000000, -0.8571428571428567622 ) ) ;
#19698=ORIENTED_EDGE ( 'NONE', *, *, #208, .T. ) ;
#19701=ORIENTED_EDGE ( 'NONE', *, *, #19412, .T. ) ;
#19713=CIRCLE ( 'NONE', #17831, 2.549999999999997158 ) ;
#19722=CARTESIAN_POINT ( 'NONE',  ( -7.518994333257361440, -2.258039616118830750, 8.837702940568419763 ) ) ;
#19741=DIRECTION ( 'NONE',  ( 1.000000000000000000, 2.891205793294682764E-16, 0.000000000000000000 ) ) ;
#19760=CARTESIAN_POINT ( 'NONE',  ( 8.079084010241055935, -11.97965595983265352, 6.665520415301795509 ) ) ;
#19764=AXIS2_PLACEMENT_3D ( 'NONE', #1336, #17309, #19323 ) ;
#19765=DIRECTION ( 'NONE',  ( 1.000000000000000000, 4.252453317207022894E-31, -5.551115123125818447E-17 ) ) ;
#19768=CARTESIAN_POINT ( 'NONE',  ( -8.697224362268011433, -14.00000000000004441, 6.250000000000033751 ) ) ;
#19770=CARTESIAN_POINT ( 'NONE',  ( 8.165409815605466193, -2.008174044758946231, 6.581206704444427125 ) ) ;
#19777=ORIENTED_EDGE ( 'NONE', *, *, #4454, .F. ) ;
#19787=CARTESIAN_POINT ( 'NONE',  ( 7.854293383767760872, -11.68772904158814008, 7.820081954006964153 ) ) ;
#19788=CARTESIAN_POINT ( 'NONE',  ( -7.576750937466543157, -11.88724926130080028, 7.200086239788027420 ) ) ;
#19789=DIRECTION ( 'NONE',  ( 0.000000000000000000, 0.000000000000000000, -1.000000000000000000 ) ) ;
#19791=ADVANCED_FACE ( 'NONE', ( #2363 ), #925, .T. ) ;
#19795=CARTESIAN_POINT ( 'NONE',  ( 6.999999999999978684, -3.018576030000261312, 8.916666666666724694 ) ) ;
#19836=CIRCLE ( 'NONE', #9689, 0.4999999999999995559 ) ;
#19857=CARTESIAN_POINT ( 'NONE',  ( 8.495599073428120818, -1.515757017040944898, 7.013360899078348254 ) ) ;
#19860=CARTESIAN_POINT ( 'NONE',  ( 10.50000000000000888, -13.50000000000003020, 5.750000000000060396 ) ) ;
#19868=AXIS2_PLACEMENT_3D ( 'NONE', #8340, #6351, #13525 ) ;
#19872=CARTESIAN_POINT ( 'NONE',  ( -10.49999999999995381, -2.000000000000005329, 9.249999999999966249 ) ) ;
#19885=CARTESIAN_POINT ( 'NONE',  ( 7.499999999999978684, -12.60977222864647196, 9.250000000000087041 ) ) ;
#19891=ADVANCED_FACE ( 'NONE', ( #2706 ), #1085, .F. ) ;
#19896=AXIS2_PLACEMENT_3D ( 'NONE', #4095, #19011, #11826 ) ;
#19897=ORIENTED_EDGE ( 'NONE', *, *, #23225, .T. ) ;
#19905=CARTESIAN_POINT ( 'NONE',  ( 7.473326079327783589, -0.1514770120355188321, 7.598194856234280259 ) ) ;
#19906=CARTESIAN_POINT ( 'NONE',  ( 7.802869476033197138, -11.64353246333685021, 7.917139222843311508 ) ) ;
#19908=FACE_OUTER_BOUND ( 'NONE', #7914, .T. ) ;
#19920=CARTESIAN_POINT ( 'NONE',  ( -10.49999999999995381, -1.499999999999997780, 6.250000000000019540 ) ) ;
#19925=VERTEX_POINT ( 'NONE', #15179 ) ;
#19926=ORIENTED_EDGE ( 'NONE', *, *, #14362, .T. ) ;
#19934=CARTESIAN_POINT ( 'NONE',  ( -12.85000000000001386, -14.00000000000007105, 5.551115123125782702E-14 ) ) ;
#19948=DIRECTION ( 'NONE',  ( 0.000000000000000000, 0.000000000000000000, 1.000000000000000000 ) ) ;
#19956=ORIENTED_EDGE ( 'NONE', *, *, #12959, .F. ) ;
#19958=AXIS2_PLACEMENT_3D ( 'NONE', #9145, #16071, #16310 ) ;
#19963=DIRECTION ( 'NONE',  ( 1.454462294001240516E-30, 1.000000000000000000, 0.000000000000000000 ) ) ;
#19964=CARTESIAN_POINT ( 'NONE',  ( 12.84999999999997300, -0.5000000000000004441, -5.749999999999963585 ) ) ;
#19966=CARTESIAN_POINT ( 'NONE',  ( -8.565230440156010872, -1.999999999999984457, 6.320505311736922316 ) ) ;
#19968=CARTESIAN_POINT ( 'NONE',  ( 8.391189084741263571, -1.526797151860789903, 7.111621047081309044 ) ) ;
#19975=B_SPLINE_CURVE_WITH_KNOTS ( 'NONE', 3,
 ( #3422, #14472, #8831, #9052, #17643, #16212, #12460, #1535, #12219, #23076, #14239, #1760, #6960, #19768 ),
 .UNSPECIFIED., .F., .F.,
 ( 4, 2, 2, 2, 2, 2, 4 ),
 ( 0.000000000000000000, 0.001000930383652479713, 0.001501395575478720870, 0.002001860767304962027, 0.002502325959131202968, 0.003002791150957444342, 0.004003721534609925789 ),
 .UNSPECIFIED. ) ;
#19977=ORIENTED_EDGE ( 'NONE', *, *, #3523, .T. ) ;
#19980=EDGE_LOOP ( 'NONE', ( #3794, #4222, #22588, #780 ) ) ;
#19987=AXIS2_PLACEMENT_3D ( 'NONE', #20366, #6137, #18606 ) ;
#19990=CARTESIAN_POINT ( 'NONE',  ( 8.414481090081482151, -14.00000000000005151, 6.435353702847478985 ) ) ;
#19995=LINE ( 'NONE', #5886, #1405 ) ;
#20006=VECTOR ( 'NONE', #16068, 1000.000000000000000 ) ;
#20012=CARTESIAN_POINT ( 'NONE',  ( 7.000000000000007105, -0.7870719649792512485, 9.239863038076343571 ) ) ;
#20013=CARTESIAN_POINT ( 'NONE',  ( 7.568091547084029536, -11.30436690654924803, 8.516664522246443880 ) ) ;
#20014=DIRECTION ( 'NONE',  ( -9.121204216617949000E-31, -1.000000000000000000, 6.982962677686261977E-15 ) ) ;
#20038=EDGE_LOOP ( 'NONE', ( #18495, #22206, #19491, #13531 ) ) ;
#20040=ORIENTED_EDGE ( 'NONE', *, *, #15414, .F. ) ;
#20049=TOROIDAL_SURFACE ( 'NONE', #14031, 5.500000000000000000, 0.5000000000000000000 ) ;
#20075=EDGE_LOOP ( 'NONE', ( #19926, #21493, #15002, #8057 ) ) ;
#20076=ORIENTED_EDGE ( 'NONE', *, *, #14489, .T. ) ;
#20079=CLOSED_SHELL ( 'NONE', ( #2323, #1334, #8534, #17776, #10416, #11946, #3698, #15033, #8210, #16307, #207, #2571, #2494, #19444, #19891, #5279, #21863, #9513, #21608, #21880, #15563, #723, #14964, #18175, #17642, #2064, #8079, #15811, #11637, #3784, #15726, #20384, #4775, #15025, #10127, #9704, #5516, #22355, #13439, #3956, #12554, #898, #14133, #21742, #19791, #22053, #14941, #22533, #8592, #38, #20480, #11313, #9086, #20185, #20599, #6395, #22239, #3091, #5500, #1050, #10661, #16124, #21397, #1585, #2769, #21994, #4934, #16862, #15552, #6632, #6420, #18410, #2605, #13090, #16731, #1753, #19663, #1177, #14435, #11963, #6646, #3089, #9417, #10835, #1563, #19407 ) ) ;
#20085=DIRECTION ( 'NONE',  ( -1.000000000000000000, -6.224605580259554159E-31, 2.887593071917436153E-31 ) ) ;
#20086=CARTESIAN_POINT ( 'NONE',  ( 7.518994333257404961, -11.74196038388119767, 8.837702940568448184 ) ) ;
#20088=CARTESIAN_POINT ( 'NONE',  ( -7.499999999999978684, -5.999999999999981348, 10.74999999999998224 ) ) ;
#20104=DIRECTION ( 'NONE',  ( 1.000000000000000000, 1.910522504832140594E-31, -5.551115123125818447E-17 ) ) ;
#20124=ORIENTED_EDGE ( 'NONE', *, *, #8436, .T. ) ;
#20125=CARTESIAN_POINT ( 'NONE',  ( 12.84999999999997300, -12.00000000000005151, 2.550000000000038902 ) ) ;
#20128=CARTESIAN_POINT ( 'NONE',  ( 6.999999991928306464, -11.17450167042447617, 8.700799235122161690 ) ) ;
#20136=EDGE_CURVE ( 'NONE', #1206, #195, #16317, .T. ) ;
#20147=FACE_OUTER_BOUND ( 'NONE', #8143, .T. ) ;
#20148=VERTEX_POINT ( 'NONE', #2455 ) ;
#20158=ORIENTED_EDGE ( 'NONE', *, *, #17610, .F. ) ;
#20160=FACE_OUTER_BOUND ( 'NONE', #22359, .T. ) ;
#20168=CARTESIAN_POINT ( 'NONE',  ( -7.568091547083694692, -2.695633093451115680, 8.516664522246127689 ) ) ;
#20185=ADVANCED_FACE ( 'NONE', ( #14582 ), #404, .T. ) ;
#20191=ORIENTED_EDGE ( 'NONE', *, *, #22325, .F. ) ;
#20195=LINE ( 'NONE', #5730, #19299 ) ;
#20203=DIRECTION ( 'NONE',  ( -2.168404344971017743E-16, 1.000000000000000000, 7.722382221513089478E-47 ) ) ;
#20206=CARTESIAN_POINT ( 'NONE',  ( -7.901093513163778503, -12.32682690073933252, 7.745538272134556479 ) ) ;
#20208=CARTESIAN_POINT ( 'NONE',  ( -7.499999999999992006, -12.60977222864646485, 9.250000000000071054 ) ) ;
#20210=CARTESIAN_POINT ( 'NONE',  ( -12.85000000000002807, -12.50000000000002842, 6.250000000000061284 ) ) ;
#20217=CIRCLE ( 'NONE', #1420, 5.500000000000000000 ) ;
#20233=CARTESIAN_POINT ( 'NONE',  ( -12.85000000000001386, -12.00000000000006928, 4.163336342344337027E-14 ) ) ;
#20236=CARTESIAN_POINT ( 'NONE',  ( 7.000000000000020428, -13.21292803502076652, 9.239863038076370216 ) ) ;
#20237=CARTESIAN_POINT ( 'NONE',  ( 7.748687480237922642, -13.73110298228169590, 8.040801957829224023 ) ) ;
#20244=TOROIDAL_SURFACE ( 'NONE', #2956, 4.500000000000000888, 0.5000000000000000000 ) ;
#20252=CARTESIAN_POINT ( 'NONE',  ( 7.835312244869989229, -0.05103360697234643473, 7.041165740960562580 ) ) ;
#20261=TOROIDAL_SURFACE ( 'NONE', #10114, 5.750000000000000000, 0.5000000000000000000 ) ;
#20267=CARTESIAN_POINT ( 'NONE',  ( -6.999999999999992006, -8.000000000000044409, 6.250000000000019540 ) ) ;
#20281=CARTESIAN_POINT ( 'NONE',  ( 12.84999999999997300, -1.999999999999998224, 0.000000000000000000 ) ) ;
#20289=CARTESIAN_POINT ( 'NONE',  ( -12.85000000000002807, -13.50000000000003020, 6.250000000000033751 ) ) ;
#20296=ORIENTED_EDGE ( 'NONE', *, *, #3523, .F. ) ;
#20307=ORIENTED_EDGE ( 'NONE', *, *, #7782, .F. ) ;
#20309=FACE_OUTER_BOUND ( 'NONE', #7968, .T. ) ;
#20316=CARTESIAN_POINT ( 'NONE',  ( -7.602880770961808032, -11.99349919129478792, 8.461619612152084358 ) ) ;
#20318=CARTESIAN_POINT ( 'NONE',  ( -7.176407415342067608, -13.63581929081302313, 8.314790908397574398 ) ) ;
#20334=DIRECTION ( 'NONE',  ( 0.000000000000000000, 0.000000000000000000, 1.000000000000000000 ) ) ;
#20337=DIRECTION ( 'NONE',  ( -9.121204216617949000E-31, -1.000000000000000000, 6.982962677686261977E-15 ) ) ;
#20341=CARTESIAN_POINT ( 'NONE',  ( 7.490952241692768077, -13.34551170378462537, 8.992386117842924520 ) ) ;
#20366=CARTESIAN_POINT ( 'NONE',  ( -4.163336342344337027E-14, 2.081668171172168513E-14, 10.24999999999993960 ) ) ;
#20372=DIRECTION ( 'NONE',  ( -9.121204216617949000E-31, -1.000000000000000000, 6.982962677686261977E-15 ) ) ;
#20384=ADVANCED_FACE ( 'NONE', ( #4905 ), #16187, .F. ) ;
#20388=ORIENTED_EDGE ( 'NONE', *, *, #8234, .F. ) ;
#20391=ORIENTED_EDGE ( 'NONE', *, *, #6957, .T. ) ;
#20396=CARTESIAN_POINT ( 'NONE',  ( -6.999999999999978684, -10.98142396999974046, 8.916666666666724694 ) ) ;
#20404=CARTESIAN_POINT ( 'NONE',  ( 7.000000000000001776, -3.018576030000261756, 8.916666666666687391 ) ) ;
#20411=ORIENTED_EDGE ( 'NONE', *, *, #5708, .T. ) ;
#20416=VERTEX_POINT ( 'NONE', #17978 ) ;
#20419=AXIS2_PLACEMENT_3D ( 'NONE', #20515, #7800, #16494 ) ;
#20425=CARTESIAN_POINT ( 'NONE',  ( 12.85000000000001386, -13.50000000000011191, -5.749999999999949374 ) ) ;
#20435=CARTESIAN_POINT ( 'NONE',  ( -7.971461718369612370, -11.76779483280641792, 7.625732677302382356 ) ) ;
#20446=CIRCLE ( 'NONE', #2775, 6.000000000000000000 ) ;
#20452=VERTEX_POINT ( 'NONE', #15839 ) ;
#20459=DIRECTION ( 'NONE',  ( -4.014645758689187542E-14, -6.938893903907237844E-15, -1.000000000000000000 ) ) ;
#20480=ADVANCED_FACE ( 'NONE', ( #17859 ), #16073, .T. ) ;
#20484=ORIENTED_EDGE ( 'NONE', *, *, #8411, .T. ) ;
#20496=B_SPLINE_CURVE_WITH_KNOTS ( 'NONE', 3,
 ( #21492, #1377, #1826, #14188, #14305, #10650, #8777, #23015, #12526, #5368, #9011, #12051, #13943, #19722, #8544, #1715 ),
 .UNSPECIFIED., .F., .F.,
 ( 4, 2, 2, 2, 2, 2, 2, 4 ),
 ( 0.000000000000000000, 0.0004262889904590540019, 0.0008525779809181080037, 0.001278866971377162114, 0.001705155961836216007, 0.002131444952295269684, 0.002557733942754324228, 0.003410311923672431147 ),
 .UNSPECIFIED. ) ;
#20506=ORIENTED_EDGE ( 'NONE', *, *, #6222, .T. ) ;
#20509=VERTEX_POINT ( 'NONE', #5859 ) ;
#20515=CARTESIAN_POINT ( 'NONE',  ( 7.000000000000006217, -5.999999999999981348, 6.250000000000005329 ) ) ;
#20519=FACE_OUTER_BOUND ( 'NONE', #15766, .T. ) ;
#20523=DIRECTION ( 'NONE',  ( 0.8571428571428568732, 3.574076823648863958E-15, 0.5150787536377136044 ) ) ;
#20524=DIRECTION ( 'NONE',  ( 0.000000000000000000, 0.000000000000000000, 1.000000000000000000 ) ) ;
#20527=EDGE_CURVE ( 'NONE', #23124, #19457, #14816, .T. ) ;
#20533=ORIENTED_EDGE ( 'NONE', *, *, #17582, .T. ) ;
#20539=VERTEX_POINT ( 'NONE', #20088 ) ;
#20548=DIRECTION ( 'NONE',  ( -1.000000000000000000, -6.224605580259554159E-31, 2.887593071917436153E-31 ) ) ;
#20549=CARTESIAN_POINT ( 'NONE',  ( -8.518530740350131580, -11.95646899714138911, 6.984205661426534206 ) ) ;
#20550=CARTESIAN_POINT ( 'NONE',  ( -6.999999999999978684, -5.999999999999981348, 11.74999999999998224 ) ) ;
#20551=FACE_OUTER_BOUND ( 'NONE', #22854, .T. ) ;
#20555=SHAPE_REPRESENTATION_RELATIONSHIP ( 'NONE' , 'NONE' ,  #1856, #8352 ) ;
#20568=CARTESIAN_POINT ( 'NONE',  ( 12.84999999999997300, -1.999999999999998224, -2.549999999999997158 ) ) ;
#20577=DIRECTION ( 'NONE',  ( 1.000000000000000000, 4.252453317207022018E-31, -5.551115123125818447E-17 ) ) ;
#20578=CARTESIAN_POINT ( 'NONE',  ( -8.502135871254283828, -0.5075717384767730600, 6.995667647939113110 ) ) ;
#20589=VERTEX_POINT ( 'NONE', #7726 ) ;
#20599=ADVANCED_FACE ( 'NONE', ( #13024 ), #11470, .T. ) ;
#20608=CARTESIAN_POINT ( 'NONE',  ( -6.999999999999992006, -8.000000000000044409, 6.250000000000019540 ) ) ;
#20614=EDGE_CURVE ( 'NONE', #138, #9220, #17698, .T. ) ;
#20615=VECTOR ( 'NONE', #6587, 1000.000000000000000 ) ;
#20619=CARTESIAN_POINT ( 'NONE',  ( 12.84999999999997300, -1.999999999999998224, 0.000000000000000000 ) ) ;
#20620=ORIENTED_EDGE ( 'NONE', *, *, #9580, .T. ) ;
#20626=ORIENTED_EDGE ( 'NONE', *, *, #19043, .F. ) ;
#20629=VERTEX_POINT ( 'NONE', #22425 ) ;
#20635=( BOUNDED_SURFACE ( )  B_SPLINE_SURFACE ( 3, 2, ( 
 ( #11707, #22316, #8193 ),
 ( #13249, #16882, #7955 ),
 ( #911, #793, #6077 ),
 ( #15356, #16648, #20316 ),
 ( #18897, #11593, #4179 ),
 ( #22194, #22546, #11250 ),
 ( #15117, #1022, #6200 ),
 ( #6431, #20435, #20206 ),
 ( #11353, #22079, #4296 ),
 ( #4074, #13370, #9609 ),
 ( #15230, #18428, #18546 ),
 ( #2306, #20549, #4414 ),
 ( #562, #14895, #16760 ),
 ( #15008, #9839, #16990 ) ),
 .UNSPECIFIED., .F., .F., .T. ) 
 B_SPLINE_SURFACE_WITH_KNOTS ( ( 4, 2, 2, 2, 2, 2, 4 ),
 ( 3, 3 ),
 ( 2.168404344971008868E-19, 0.0009656398008937970437, 0.001448459701340695403, 0.001931279601787593871, 0.002414099502234492121, 0.002896919402681390806, 0.003862559203575187741 ),
 ( 0.000000000000000000, 1.000000000000000000 ),
 .UNSPECIFIED. ) 
 GEOMETRIC_REPRESENTATION_ITEM ( )  RATIONAL_B_SPLINE_SURFACE ( (
 ( 1.000000000000000000, 0.7071067811865499042, 1.000000000000000000),
 ( 1.000000000000000000, 0.6907538105665188555, 1.000000000000000000),
 ( 1.000000000000000000, 0.6765417438352628876, 1.000000000000000000),
 ( 1.000000000000000000, 0.6623232117677045894, 1.000000000000000000),
 ( 1.000000000000000000, 0.6588386061805797667, 1.000000000000000000),
 ( 1.000000000000000000, 0.6547992448372288443, 1.000000000000000000),
 ( 1.000000000000000000, 0.6542040191408818872, 1.000000000000000000),
 ( 1.000000000000000000, 0.6557724471762286234, 1.000000000000000000),
 ( 1.000000000000000000, 0.6579729115736443479, 1.000000000000000000),
 ( 1.000000000000000000, 0.6644691908065893937, 1.000000000000000000),
 ( 1.000000000000000000, 0.6687559023949966042, 1.000000000000000000),
 ( 1.000000000000000000, 0.6835702420292867343, 1.000000000000000000),
 ( 1.000000000000000000, 0.6960226107071281199, 1.000000000000000000),
 ( 1.000000000000000000, 0.7071067811865473507, 1.000000000000000000) ) ) 
 REPRESENTATION_ITEM ( '' )  SURFACE ( )  );
#20639=CARTESIAN_POINT ( 'NONE',  ( -8.954763739086814667, -1.999999999999985567, 6.678571428571395963 ) ) ;
#20647=CYLINDRICAL_SURFACE ( 'NONE', #22492, 0.4999999999999987232 ) ;
#20658=ORIENTED_EDGE ( 'NONE', *, *, #7266, .T. ) ;
#20660=B_SPLINE_CURVE_WITH_KNOTS ( 'NONE', 3,
 ( #7239, #19229, #9003, #10753, #8882, #22891, #3247, #16155, #12276, #3127, #23250, #7135, #14295, #21480 ),
 .UNSPECIFIED., .F., .F.,
 ( 4, 2, 2, 2, 2, 2, 4 ),
 ( 0.000000000000000000, 0.0008249779604813624800, 0.001237466940722041064, 0.001649955920962719756, 0.002062444901203395412, 0.002474933881444070418, 0.003299911841925418261 ),
 .UNSPECIFIED. ) ;
#20663=EDGE_LOOP ( 'NONE', ( #7998, #5045, #19661, #5812 ) ) ;
#20668=DIRECTION ( 'NONE',  ( 1.454462294001240516E-30, 1.000000000000000000, 7.888609052210128564E-31 ) ) ;
#20674=CARTESIAN_POINT ( 'NONE',  ( -7.345446946324452497, -13.78184793132693642, 7.860330092054036655 ) ) ;
#20680=ORIENTED_EDGE ( 'NONE', *, *, #22146, .T. ) ;
#20688=LINE ( 'NONE', #20568, #13297 ) ;
#20692=LINE ( 'NONE', #8452, #17527 ) ;
#20705=CIRCLE ( 'NONE', #18069, 4.500000000000000888 ) ;
#20711=ORIENTED_EDGE ( 'NONE', *, *, #4473, .T. ) ;
#20715=ORIENTED_EDGE ( 'NONE', *, *, #14362, .F. ) ;
#20717=AXIS2_PLACEMENT_3D ( 'NONE', #7164, #14322, #19263 ) ;
#20722=CARTESIAN_POINT ( 'NONE',  ( -12.84999999999999964, -13.50000000000011191, -5.749999999999949374 ) ) ;
#20727=DIRECTION ( 'NONE',  ( -1.000000000000000000, -6.224605580259554159E-31, 2.887593071917436153E-31 ) ) ;
#20732=CARTESIAN_POINT ( 'NONE',  ( 6.999999999999978684, -8.000000000000031974, 10.24999999999998224 ) ) ;
#20738=ORIENTED_EDGE ( 'NONE', *, *, #9103, .T. ) ;
#20752=CARTESIAN_POINT ( 'NONE',  ( -7.324400034341836729, -2.232976452217596997, 7.601326208249630234 ) ) ;
#20756=CARTESIAN_POINT ( 'NONE',  ( 7.263517083688649123, -2.279413854694211761, 7.724990489865469989 ) ) ;
#20761=AXIS2_PLACEMENT_3D ( 'NONE', #7271, #14087, #7159 ) ;
#20776=VERTEX_POINT ( 'NONE', #7778 ) ;
#20780=AXIS2_PLACEMENT_3D ( 'NONE', #4256, #16726, #5702 ) ;
#20785=ORIENTED_EDGE ( 'NONE', *, *, #8539, .T. ) ;
#20790=B_SPLINE_CURVE_WITH_KNOTS ( 'NONE', 3,
 ( #3440, #14492, #17909, #6986, #5556, #3561, #18029, #19788, #18251, #1784, #10942, #3774, #2010, #41 ),
 .UNSPECIFIED., .F., .F.,
 ( 4, 2, 2, 2, 2, 2, 4 ),
 ( 0.000000000000000000, 0.0004465115319127595738, 0.0008930230638255191476, 0.001339534595738282570, 0.001786046127651045885, 0.002679069191476572079, 0.003572092255302097407 ),
 .UNSPECIFIED. ) ;
#20794=CARTESIAN_POINT ( 'NONE',  ( -7.991520206789724412, -13.39565235458639059, 7.599114430427917455 ) ) ;
#20805=DIRECTION ( 'NONE',  ( -9.121204216617949000E-31, -1.000000000000000000, 6.982962677686261977E-15 ) ) ;
#20823=DIRECTION ( 'NONE',  ( -9.121204216617949000E-31, -1.000000000000000000, 6.982962677686261977E-15 ) ) ;
#20825=CARTESIAN_POINT ( 'NONE',  ( -7.694134585029414275, -0.3119908745746264866, 8.172315317061135787 ) ) ;
#20827=CARTESIAN_POINT ( 'NONE',  ( 8.721922330812452273, -13.98762810781384403, 6.818491697977837163 ) ) ;
#20853=DIRECTION ( 'NONE',  ( -2.753132232808523448E-17, 0.6666666666666727359, 0.7453559924999245689 ) ) ;
#20862=ORIENTED_EDGE ( 'NONE', *, *, #8067, .F. ) ;
#20870=CARTESIAN_POINT ( 'NONE',  ( -7.971461718369176275, -2.232205167193757056, 7.625732677302567986 ) ) ;
#20881=PRODUCT_DEFINITION_CONTEXT ( 'detailed design', #18699, 'design' ) ;
#20883=ORIENTED_EDGE ( 'NONE', *, *, #17284, .T. ) ;
#20892=DIRECTION ( 'NONE',  ( 0.000000000000000000, -7.888609052210128564E-31, 1.000000000000000000 ) ) ;
#20893=ORIENTED_EDGE ( 'NONE', *, *, #17828, .F. ) ;
#20906=EDGE_CURVE ( 'NONE', #14484, #1201, #9664, .T. ) ;
#20916=ORIENTED_EDGE ( 'NONE', *, *, #2302, .F. ) ;
#20930=CARTESIAN_POINT ( 'NONE',  ( -8.954763739086819996, 1.387778780781445833E-14, 6.678571428571393298 ) ) ;
#20934=CARTESIAN_POINT ( 'NONE',  ( 12.84999999999997300, -2.000000000000001776, 6.250000000000005329 ) ) ;
#20952=DIRECTION ( 'NONE',  ( 0.000000000000000000, -7.888609052210128564E-31, 1.000000000000000000 ) ) ;
#20961=LINE ( 'NONE', #11999, #23247 ) ;
#20968=VERTEX_POINT ( 'NONE', #2959 ) ;
#20976=DIRECTION ( 'NONE',  ( -2.289258728441392898E-17, -0.5454545454545509653, -0.8381404052084406864 ) ) ;
#20977=CARTESIAN_POINT ( 'NONE',  ( -12.84999999999999964, -0.5000000000000038858, 5.750000000000018652 ) ) ;
#20979=CARTESIAN_POINT ( 'NONE',  ( -8.165409815605727317, -2.008174044758924026, 6.581206704444227285 ) ) ;
#20989=CARTESIAN_POINT ( 'NONE',  ( -8.391189084741235149, -12.47320284813923585, 7.111621047081351676 ) ) ;
#20990=DIRECTION ( 'NONE',  ( 0.000000000000000000, 6.802837160693368935E-15, 1.000000000000000000 ) ) ;
#20992=CYLINDRICAL_SURFACE ( 'NONE', #21686, 0.4999999999999995559 ) ;
#20998=ORIENTED_EDGE ( 'NONE', *, *, #6090, .T. ) ;
#21004=CYLINDRICAL_SURFACE ( 'NONE', #18147, 5.999999999999991118 ) ;
#21022=( NAMED_UNIT ( * ) SI_UNIT ( $, .STERADIAN. ) SOLID_ANGLE_UNIT ( ) );
#21032=EDGE_LOOP ( 'NONE', ( #9913, #16166 ) ) ;
#21043=CARTESIAN_POINT ( 'NONE',  ( -7.796097383573730610, -0.6999727310043959427, 7.943830786858171678 ) ) ;
#21053=ORIENTED_EDGE ( 'NONE', *, *, #19181, .F. ) ;
#21059=VERTEX_POINT ( 'NONE', #8713 ) ;
#21060=EDGE_LOOP ( 'NONE', ( #7120, #10745, #5237, #6562 ) ) ;
#21071=DIRECTION ( 'NONE',  ( 1.000000000000000000, 2.168404344970994323E-16, -1.780660105995169760E-30 ) ) ;
#21072=VECTOR ( 'NONE', #6830, 1000.000000000000000 ) ;
#21078=EDGE_CURVE ( 'NONE', #138, #20968, #19995, .T. ) ;
#21103=CARTESIAN_POINT ( 'NONE',  ( -7.518994333257403184, -11.74196038388118879, 8.837702940568457066 ) ) ;
#21107=FACE_OUTER_BOUND ( 'NONE', #1574, .T. ) ;
#21108=EDGE_CURVE ( 'NONE', #396, #14530, #12941, .T. ) ;
#21109=VERTEX_POINT ( 'NONE', #16790 ) ;
#21121=AXIS2_PLACEMENT_3D ( 'NONE', #11589, #20668, #15225 ) ;
#21128=CARTESIAN_POINT ( 'NONE',  ( -8.223343937052021602, -0.5454750081368713310, 7.291631794411020273 ) ) ;
#21131=MANIFOLD_SOLID_BREP ( 'Fillet3', #20079 ) ;
#21134=CARTESIAN_POINT ( 'NONE',  ( 7.499999999999992895, -5.999999999999967137, 10.74999999999998224 ) ) ;
#21137=LINE ( 'NONE', #21384, #1840 ) ;
#21144=AXIS2_PLACEMENT_3D ( 'NONE', #19934, #3803, #12186 ) ;
#21146=ORIENTED_EDGE ( 'NONE', *, *, #9248, .F. ) ;
#21165=CARTESIAN_POINT ( 'NONE',  ( 7.499999999999976907, -2.439868446130579294, 9.052558787159759035 ) ) ;
#21176=AXIS2_PLACEMENT_3D ( 'NONE', #11635, #6363, #22948 ) ;
#21199=CARTESIAN_POINT ( 'NONE',  ( -10.49999999999995381, -2.000000000000005329, 9.249999999999966249 ) ) ;
#21233=CARTESIAN_POINT ( 'NONE',  ( -8.200527591913225223, -12.43937801162580925, 7.318116290495828125 ) ) ;
#21251=DIRECTION ( 'NONE',  ( 1.000000000000000000, 6.224605580259554159E-31, -2.887593071917436153E-31 ) ) ;
#21253=DIRECTION ( 'NONE',  ( -1.577021341797097314E-16, 1.000000000000000000, 0.000000000000000000 ) ) ;
#21254=CARTESIAN_POINT ( 'NONE',  ( -7.980290731945666849, -0.6082991440336598110, 7.616182555102755991 ) ) ;
#21259=CARTESIAN_POINT ( 'NONE',  ( 12.84999999999997300, -0.5000000000000004441, 1.387778780781445676E-14 ) ) ;
#21263=DIRECTION ( 'NONE',  ( -0.8571428571428572063, -2.366582715663038569E-30, 0.5150787536377126052 ) ) ;
#21264=DIRECTION ( 'NONE',  ( -2.289258728441392898E-17, -0.5454545454545509653, -0.8381404052084407974 ) ) ;
#21268=ORIENTED_EDGE ( 'NONE', *, *, #20614, .T. ) ;
#21276=CARTESIAN_POINT ( 'NONE',  ( -7.991520206789717307, -0.6043476454136054166, 7.599114430427804656 ) ) ;
#21281=CARTESIAN_POINT ( 'NONE',  ( 7.713464495932033316, -1.828647720521569875, 8.131426806228642334 ) ) ;
#21282=CARTESIAN_POINT ( 'NONE',  ( -7.500000000000020428, -12.00000000000002132, 9.250000000000008882 ) ) ;
#21286=ORIENTED_EDGE ( 'NONE', *, *, #3516, .T. ) ;
#21287=ORIENTED_EDGE ( 'NONE', *, *, #6090, .F. ) ;
#21300=ORIENTED_EDGE ( 'NONE', *, *, #15183, .F. ) ;
#21302=CARTESIAN_POINT ( 'NONE',  ( 6.999999999999992006, -5.999999999999981348, 12.25000000000001066 ) ) ;
#21303=CARTESIAN_POINT ( 'NONE',  ( -12.85000000000005649, -12.00000000000011191, -6.249999999999936051 ) ) ;
#21322=VERTEX_POINT ( 'NONE', #21638 ) ;
#21325=AXIS2_PLACEMENT_3D ( 'NONE', #11569, #4275, #21747 ) ;
#21331=CYLINDRICAL_SURFACE ( 'NONE', #18471, 2.549999999999997158 ) ;
#21335=EDGE_CURVE ( 'NONE', #19516, #16622, #10006, .T. ) ;
#21341=FACE_BOUND ( 'NONE', #19459, .T. ) ;
#21343=AXIS2_PLACEMENT_3D ( 'NONE', #20233, #16446, #11498 ) ;
#21355=AXIS2_PLACEMENT_3D ( 'NONE', #2815, #9992, #6457 ) ;
#21358=EDGE_CURVE ( 'NONE', #9332, #6633, #11023, .T. ) ;
#21359=AXIS2_PLACEMENT_3D ( 'NONE', #13947, #21264, #16053 ) ;
#21384=CARTESIAN_POINT ( 'NONE',  ( -12.84999999999999964, -6.938893903907228378E-15, 5.749999999999991118 ) ) ;
#21385=TOROIDAL_SURFACE ( 'NONE', #21325, 3.500000000000000000, 0.5000000000000000000 ) ;
#21389=ORIENTED_EDGE ( 'NONE', *, *, #19000, .T. ) ;
#21396=CARTESIAN_POINT ( 'NONE',  ( 8.223343937052055352, -0.5454750081368732184, 7.291631794411076228 ) ) ;
#21397=ADVANCED_FACE ( 'NONE', ( #2312 ), #4080, .T. ) ;
#21400=CIRCLE ( 'NONE', #10859, 0.4999999999999999445 ) ;
#21414=EDGE_CURVE ( 'NONE', #12422, #9827, #16741, .T. ) ;
#21433=CARTESIAN_POINT ( 'NONE',  ( 8.719386969281730515, -1.499999991380386533, 6.820015264002347699 ) ) ;
#21437=DIRECTION ( 'NONE',  ( -1.000000000000000000, -6.224605580259554159E-31, 2.887593071917436153E-31 ) ) ;
#21447=LINE ( 'NONE', #16229, #9885 ) ;
#21450=CARTESIAN_POINT ( 'NONE',  ( 7.324400034341882026, -11.76702354778242920, 7.601326208249671978 ) ) ;
#21453=CARTESIAN_POINT ( 'NONE',  ( -8.414481090081508796, 1.743352624126960279E-14, 6.435353702847428359 ) ) ;
#21461=LINE ( 'NONE', #5097, #8574 ) ;
#21462=CARTESIAN_POINT ( 'NONE',  ( 7.268749084027611218, -2.258953384213798987, 7.689023314178105473 ) ) ;
#21480=CARTESIAN_POINT ( 'NONE',  ( -7.500000000000034639, -12.60977222864646485, 9.250000000000063949 ) ) ;
#21483=CARTESIAN_POINT ( 'NONE',  ( 12.84999999999997300, 0.000000000000000000, 1.387778780781445676E-14 ) ) ;
#21491=LINE ( 'NONE', #21134, #17811 ) ;
#21492=CARTESIAN_POINT ( 'NONE',  ( -8.954763739086851970, -1.500000000000001332, 6.678571428571422608 ) ) ;
#21493=ORIENTED_EDGE ( 'NONE', *, *, #5708, .F. ) ;
#21497=ORIENTED_EDGE ( 'NONE', *, *, #20527, .T. ) ;
#21507=DIRECTION ( 'NONE',  ( -1.000000000000000000, -1.910522504832140594E-31, 5.551115123125818447E-17 ) ) ;
#21527=FACE_OUTER_BOUND ( 'NONE', #5234, .T. ) ;
#21533=CIRCLE ( 'NONE', #479, 2.549999999999997158 ) ;
#21535=CARTESIAN_POINT ( 'NONE',  ( 7.268749084027636975, -11.74104661578624409, 7.689023314178095703 ) ) ;
#21558=ORIENTED_EDGE ( 'NONE', *, *, #14489, .F. ) ;
#21559=ORIENTED_EDGE ( 'NONE', *, *, #7772, .T. ) ;
#21561=CARTESIAN_POINT ( 'NONE',  ( 7.735962016526126916, -0.06991241830943736857, 7.174192622767028737 ) ) ;
#21568=AXIS2_PLACEMENT_3D ( 'NONE', #8697, #6699, #19391 ) ;
#21569=CARTESIAN_POINT ( 'NONE',  ( 8.954763739086866181, -13.50000000000002309, 6.678571428571478563 ) ) ;
#21575=CARTESIAN_POINT ( 'NONE',  ( 12.84999999999997300, -2.000000000000001776, 5.749999999999976907 ) ) ;
#21579=CARTESIAN_POINT ( 'NONE',  ( 7.500000000000006217, -1.217419751680345108, 9.022398393216416679 ) ) ;
#21588=ORIENTED_EDGE ( 'NONE', *, *, #19156, .F. ) ;
#21600=VECTOR ( 'NONE', #13335, 1000.000000000000000 ) ;
#21601=TOROIDAL_SURFACE ( 'NONE', #6936, 3.500000000000000000, 0.5000000000000000000 ) ;
#21602=DIRECTION ( 'NONE',  ( 0.000000000000000000, 0.000000000000000000, -1.000000000000000000 ) ) ;
#21607=ORIENTED_EDGE ( 'NONE', *, *, #12975, .T. ) ;
#21608=ADVANCED_FACE ( 'NONE', ( #2896 ), #1147, .F. ) ;
#21621=CARTESIAN_POINT ( 'NONE',  ( 6.999999999999978684, -5.999999999999981348, 11.74999999999998224 ) ) ;
#21624=CARTESIAN_POINT ( 'NONE',  ( 10.49999999999998224, 0.000000000000000000, 5.750000000000005329 ) ) ;
#21625=DIRECTION ( 'NONE',  ( 1.454462294001240516E-30, 1.000000000000000000, 0.000000000000000000 ) ) ;
#21631=CARTESIAN_POINT ( 'NONE',  ( -7.568268608012067133, -13.53268520232740357, 8.579161250779877790 ) ) ;
#21638=CARTESIAN_POINT ( 'NONE',  ( 8.954763739086851970, -1.500000000000001332, 6.678571428571422608 ) ) ;
#21643=EDGE_CURVE ( 'NONE', #3351, #20629, #20496, .T. ) ;
#21649=CARTESIAN_POINT ( 'NONE',  ( 8.697224362267997222, -12.00000000000002842, 6.250000000000019540 ) ) ;
#21675=CARTESIAN_POINT ( 'NONE',  ( 7.523705677365021494, -11.16164950473969775, 8.715168381946160281 ) ) ;
#21676=CARTESIAN_POINT ( 'NONE',  ( -12.84999999999999964, -12.50000000000006928, 6.938893903907228378E-14 ) ) ;
#21686=AXIS2_PLACEMENT_3D ( 'NONE', #15905, #8515, #3349 ) ;
#21691=CARTESIAN_POINT ( 'NONE',  ( 8.510464245293309915, -0.5071972189929013775, 6.988717072694006660 ) ) ;
#21694=ORIENTED_EDGE ( 'NONE', *, *, #7359, .F. ) ;
#21699=ORIENTED_EDGE ( 'NONE', *, *, #21108, .F. ) ;
#21701=AXIS2_PLACEMENT_3D ( 'NONE', #14456, #1517, #5041 ) ;
#21702=EDGE_LOOP ( 'NONE', ( #2648, #3747, #8003, #17688 ) ) ;
#21715=FACE_OUTER_BOUND ( 'NONE', #10543, .T. ) ;
#21737=CARTESIAN_POINT ( 'NONE',  ( 8.391189084741249360, -12.47320284813923585, 7.111621047081361446 ) ) ;
#21739=CARTESIAN_POINT ( 'NONE',  ( -8.697224362267997222, -1.999999999999998224, 6.249999999999977796 ) ) ;
#21742=ADVANCED_FACE ( 'NONE', ( #300 ), #14902, .T. ) ;
#21747=DIRECTION ( 'NONE',  ( -4.019602852144232182E-47, -6.982962677686261977E-15, -1.000000000000000000 ) ) ;
#21749=EDGE_CURVE ( 'NONE', #17392, #11726, #10025, .T. ) ;
#21769=CARTESIAN_POINT ( 'NONE',  ( 7.604097569491849562, -13.58924811263090326, 8.440516644273110103 ) ) ;
#21779=SHAPE_DEFINITION_REPRESENTATION ( #4390, #1856 ) ;
#21784=ORIENTED_EDGE ( 'NONE', *, *, #15556, .F. ) ;
#21790=CARTESIAN_POINT ( 'NONE',  ( 7.901093513163756299, -12.32682690073933252, 7.745538272134628421 ) ) ;
#21804=CARTESIAN_POINT ( 'NONE',  ( 7.761744141695581689, -2.064358047808337204, 6.973942750959555958 ) ) ;
#21824=LINE ( 'NONE', #5710, #13633 ) ;
#21835=ORIENTED_EDGE ( 'NONE', *, *, #6624, .F. ) ;
#21846=CARTESIAN_POINT ( 'NONE',  ( 8.715898959466901630, -12.49756837761076333, 6.833978265954070430 ) ) ;
#21850=CARTESIAN_POINT ( 'NONE',  ( -10.49999999999998224, -14.00000000000003020, 6.250000000000033751 ) ) ;
#21863=ADVANCED_FACE ( 'NONE', ( #18758 ), #7933, .F. ) ;
#21880=ADVANCED_FACE ( 'NONE', ( #6181 ), #15091, .F. ) ;
#21888=VECTOR ( 'NONE', #6096, 1000.000000000000000 ) ;
#21889=ORIENTED_EDGE ( 'NONE', *, *, #11979, .T. ) ;
#21895=CARTESIAN_POINT ( 'NONE',  ( 7.126417736726676999, -0.4330224014298832969, 8.494066294656319016 ) ) ;
#21896=CARTESIAN_POINT ( 'NONE',  ( 8.260108127873353467, -11.89083139210928408, 7.249251683976535077 ) ) ;
#21897=ORIENTED_EDGE ( 'NONE', *, *, #7266, .F. ) ;
#21906=FACE_OUTER_BOUND ( 'NONE', #22656, .T. ) ;
#21918=CARTESIAN_POINT ( 'NONE',  ( 8.496394830447160373, -0.03251735406450768917, 6.998792816380077220 ) ) ;
#21919=VERTEX_POINT ( 'NONE', #15447 ) ;
#21920=EDGE_LOOP ( 'NONE', ( #17654, #7912, #8698, #8634 ) ) ;
#21929=AXIS2_PLACEMENT_3D ( 'NONE', #18182, #2051, #19587 ) ;
#21942=CARTESIAN_POINT ( 'NONE',  ( -7.710998176012503258, -2.456120859166647019, 8.114728912742579681 ) ) ;
#21946=DIRECTION ( 'NONE',  ( 0.000000000000000000, 3.469446951953619316E-15, 1.000000000000000000 ) ) ;
#21957=EDGE_LOOP ( 'NONE', ( #1570, #12766 ) ) ;
#21972=CARTESIAN_POINT ( 'NONE',  ( 8.200527591913257197, -1.560621988374212732, 7.318116290495780163 ) ) ;
#21980=ORIENTED_EDGE ( 'NONE', *, *, #18700, .T. ) ;
#21981=CARTESIAN_POINT ( 'NONE',  ( 12.84999999999997300, -12.00000000000005151, 2.550000000000038902 ) ) ;
#21983=EDGE_LOOP ( 'NONE', ( #16666, #19897, #13095, #7789 ) ) ;
#21994=ADVANCED_FACE ( 'NONE', ( #21107 ), #20992, .T. ) ;
#21995=CARTESIAN_POINT ( 'NONE',  ( 7.499999999999976019, -12.78258024831459139, 9.022398393212654355 ) ) ;
#22010=ORIENTED_EDGE ( 'NONE', *, *, #12002, .F. ) ;
#22011=DIRECTION ( 'NONE',  ( 2.168404344971004924E-16, 1.000000000000000000, 5.217794476051303021E-47 ) ) ;
#22012=CYLINDRICAL_SURFACE ( 'NONE', #22563, 0.4999999999999995559 ) ;
#22023=CARTESIAN_POINT ( 'NONE',  ( 7.573440241539877604, -0.1138337924791416322, 7.421600184846412596 ) ) ;
#22037=ORIENTED_EDGE ( 'NONE', *, *, #2196, .F. ) ;
#22048=AXIS2_PLACEMENT_3D ( 'NONE', #6523, #13350, #9705 ) ;
#22052=CIRCLE ( 'NONE', #10775, 6.249999999999992006 ) ;
#22053=ADVANCED_FACE ( 'NONE', ( #20147 ), #3563, .T. ) ;
#22057=CARTESIAN_POINT ( 'NONE',  ( 7.000000000000006217, -2.645898033750298417, 9.250000000000021316 ) ) ;
#22070=VECTOR ( 'NONE', #15267, 1000.000000000000000 ) ;
#22071=DIRECTION ( 'NONE',  ( -1.000000000000000000, 2.168404344971005170E-16, -1.203141491611682442E-30 ) ) ;
#22072=EDGE_LOOP ( 'NONE', ( #22010, #13183, #5850, #17934 ) ) ;
#22079=CARTESIAN_POINT ( 'NONE',  ( -8.037202331403117128, -11.80340871766187405, 7.528743044528739325 ) ) ;
#22081=CARTESIAN_POINT ( 'NONE',  ( -7.576750937466491642, -2.112750738699229469, 7.200086239787990117 ) ) ;
#22099=CARTESIAN_POINT ( 'NONE',  ( 12.84999999999997300, -1.999999999999998224, 2.549999999999997158 ) ) ;
#22109=CARTESIAN_POINT ( 'NONE',  ( 7.951003271401684280, -13.83829779185628794, 7.659883344695716190 ) ) ;
#22114=EDGE_CURVE ( 'NONE', #11691, #20589, #16937, .T. ) ;
#22115=AXIS2_PLACEMENT_3D ( 'NONE', #4943, #2963, #5306 ) ;
#22125=ORIENTED_EDGE ( 'NONE', *, *, #9147, .F. ) ;
#22132=DIRECTION ( 'NONE',  ( 2.168404344971004924E-16, 1.000000000000000000, 5.217794476051303021E-47 ) ) ;
#22135=DIRECTION ( 'NONE',  ( 0.000000000000000000, 0.000000000000000000, 1.000000000000000000 ) ) ;
#22139=DIRECTION ( 'NONE',  ( -9.121204216617949000E-31, -1.000000000000000000, 6.982962677686261977E-15 ) ) ;
#22146=EDGE_CURVE ( 'NONE', #6727, #280, #22430, .T. ) ;
#22188=ORIENTED_EDGE ( 'NONE', *, *, #15859, .F. ) ;
#22194=CARTESIAN_POINT ( 'NONE',  ( -7.263517083688649123, -11.72058614530575049, 7.724990489865638743 ) ) ;
#22201=EDGE_CURVE ( 'NONE', #13412, #5493, #14914, .T. ) ;
#22206=ORIENTED_EDGE ( 'NONE', *, *, #2789, .T. ) ;
#22232=ORIENTED_EDGE ( 'NONE', *, *, #6698, .T. ) ;
#22239=ADVANCED_FACE ( 'NONE', ( #2374 ), #2897, .T. ) ;
#22256=AXIS2_PLACEMENT_3D ( 'NONE', #6336, #810, #13741 ) ;
#22279=DIRECTION ( 'NONE',  ( 0.000000000000000000, -6.938893903907238633E-15, -1.000000000000000000 ) ) ;
#22280=CARTESIAN_POINT ( 'NONE',  ( 7.024848138040876044, -2.659619850263452268, 8.468562630484324671 ) ) ;
#22300=EDGE_LOOP ( 'NONE', ( #2518, #21287, #10717, #6839 ) ) ;
#22316=CARTESIAN_POINT ( 'NONE',  ( -7.500000000000030198, -10.98142396999974935, 8.916666666666721142 ) ) ;
#22320=CARTESIAN_POINT ( 'NONE',  ( -7.499999999999965361, -1.999999999999991340, 6.249999999999950262 ) ) ;
#22324=DIRECTION ( 'NONE',  ( -2.168404344971017743E-16, 1.000000000000000000, 1.287063703585503763E-46 ) ) ;
#22325=EDGE_CURVE ( 'NONE', #9370, #7710, #12203, .T. ) ;
#22329=VERTEX_POINT ( 'NONE', #7171 ) ;
#22338=EDGE_CURVE ( 'NONE', #1155, #6633, #17955, .T. ) ;
#22340=EDGE_CURVE ( 'NONE', #9827, #9220, #12677, .T. ) ;
#22346=CARTESIAN_POINT ( 'NONE',  ( -8.718376657154840004, -0.4999999999999867883, 6.820622386031956808 ) ) ;
#22355=ADVANCED_FACE ( 'NONE', ( #7286 ), #23052, .F. ) ;
#22359=EDGE_LOOP ( 'NONE', ( #8141, #18412, #10487, #9481 ) ) ;
#22361=EDGE_LOOP ( 'NONE', ( #23174, #20388, #15022, #21699 ) ) ;
#22366=CARTESIAN_POINT ( 'NONE',  ( 8.954763739086835983, -12.00000000000003908, 6.678571428571491886 ) ) ;
#22388=ORIENTED_EDGE ( 'NONE', *, *, #21358, .F. ) ;
#22390=EDGE_CURVE ( 'NONE', #13674, #9332, #16778, .T. ) ;
#22398=CARTESIAN_POINT ( 'NONE',  ( 7.551224464536185899, -2.121331013966567092, 7.234820221745167146 ) ) ;
#22399=CARTESIAN_POINT ( 'NONE',  ( -12.84999999999999964, -14.00000000000011369, -5.749999999999949374 ) ) ;
#22413=AXIS2_PLACEMENT_3D ( 'NONE', #22057, #13003, #11108 ) ;
#22425=CARTESIAN_POINT ( 'NONE',  ( -7.500000000000007105, -2.645898033750305522, 9.250000000000035527 ) ) ;
#22428=CARTESIAN_POINT ( 'NONE',  ( 12.84999999999997300, -1.999999999999998224, 2.549999999999997158 ) ) ;
#22430=CIRCLE ( 'NONE', #7045, 5.749999999999992006 ) ;
#22434=FACE_OUTER_BOUND ( 'NONE', #17931, .T. ) ;
#22448=TOROIDAL_SURFACE ( 'NONE', #15299, 5.500000000000000000, 0.5000000000000000000 ) ;
#22465=DIRECTION ( 'NONE',  ( -0.5150787536377109399, 0.000000000000000000, 0.8571428571428583165 ) ) ;
#22471=ORIENTED_EDGE ( 'NONE', *, *, #11545, .T. ) ;
#22477=DIRECTION ( 'NONE',  ( 2.168404344971005170E-16, 1.000000000000000000, -8.696324126752285467E-47 ) ) ;
#22492=AXIS2_PLACEMENT_3D ( 'NONE', #18635, #13463, #17087 ) ;
#22502=COLOUR_RGB ( '', 0.72549020, 0.75294118, 0.79215686) ;
#22515=CARTESIAN_POINT ( 'NONE',  ( 7.500000000000006217, -2.428697021684863788, 9.041853041249359180 ) ) ;
#22527=ORIENTED_EDGE ( 'NONE', *, *, #8205, .T. ) ;
#22533=ADVANCED_FACE ( 'NONE', ( #22434 ), #22448, .T. ) ;
#22538=ORIENTED_EDGE ( 'NONE', *, *, #1601, .T. ) ;
#22546=CARTESIAN_POINT ( 'NONE',  ( -7.802869476033403195, -11.64353246333686265, 7.917139222843291968 ) ) ;
#22547=CARTESIAN_POINT ( 'NONE',  ( -7.920269128372687817, -13.36773923605932168, 7.713069291591535759 ) ) ;
#22555=DIRECTION ( 'NONE',  ( 0.000000000000000000, 0.000000000000000000, -1.000000000000000000 ) ) ;
#22563=AXIS2_PLACEMENT_3D ( 'NONE', #16576, #7436, #19789 ) ;
#22566=LINE ( 'NONE', #6451, #17736 ) ;
#22569=CARTESIAN_POINT ( 'NONE',  ( -7.756475484083187766, -0.06559517125032440776, 7.145789564688667994 ) ) ;
#22585=DIRECTION ( 'NONE',  ( 1.000000000000000000, -2.168404344971005170E-16, 1.203141491611682442E-30 ) ) ;
#22588=ORIENTED_EDGE ( 'NONE', *, *, #3610, .F. ) ;
#22600=EDGE_CURVE ( 'NONE', #16375, #9602, #22818, .T. ) ;
#22611=EDGE_CURVE ( 'NONE', #4863, #10470, #18317, .T. ) ;
#22613=VERTEX_POINT ( 'NONE', #1266 ) ;
#22627=CARTESIAN_POINT ( 'NONE',  ( 7.324400034341884691, -2.232976452217586782, 7.601326208249607141 ) ) ;
#22636=DIRECTION ( 'NONE',  ( -1.000000000000000000, -2.168404344971017743E-16, 1.780660105995169760E-30 ) ) ;
#22643=ORIENTED_EDGE ( 'NONE', *, *, #3061, .T. ) ;
#22651=ORIENTED_EDGE ( 'NONE', *, *, #13683, .F. ) ;
#22656=EDGE_LOOP ( 'NONE', ( #11926, #17930, #20626, #21389 ) ) ;
#22667=CARTESIAN_POINT ( 'NONE',  ( -7.499999999999992895, -8.000000000000044409, 6.250000000000005329 ) ) ;
#22674=( LENGTH_UNIT ( ) NAMED_UNIT ( * ) SI_UNIT ( .MILLI., .METRE. ) );
#22681=VERTEX_POINT ( 'NONE', #3602 ) ;
#22685=VECTOR ( 'NONE', #5977, 1000.000000000000000 ) ;
#22703=VECTOR ( 'NONE', #12764, 1000.000000000000000 ) ;
#22722=CARTESIAN_POINT ( 'NONE',  ( -12.84999999999998721, -1.999999999999998224, -5.749999999999991118 ) ) ;
#22729=VECTOR ( 'NONE', #37, 1000.000000000000000 ) ;
#22736=ORIENTED_EDGE ( 'NONE', *, *, #15859, .T. ) ;
#22740=EDGE_CURVE ( 'NONE', #16729, #8301, #7083, .T. ) ;
#22741=DIRECTION ( 'NONE',  ( 1.454462294001240516E-30, 1.000000000000000000, 0.000000000000000000 ) ) ;
#22743=CARTESIAN_POINT ( 'NONE',  ( -8.260108127873330375, -2.109168607890870906, 7.249251683976359217 ) ) ;
#22754=CARTESIAN_POINT ( 'NONE',  ( -7.713464495932024434, -12.17135227947844278, 8.131426806228684967 ) ) ;
#22758=AXIS2_PLACEMENT_3D ( 'NONE', #20722, #17168, #13426 ) ;
#22773=STYLED_ITEM ( 'NONE', ( #469 ), #21131 ) ;
#22776=CARTESIAN_POINT ( 'NONE',  ( 6.999999999999992006, -8.000000000000003553, 12.25000000000001066 ) ) ;
#22783=DIRECTION ( 'NONE',  ( 1.734723475976813750E-16, 1.000000000000000000, -3.469446951953607484E-15 ) ) ;
#22786=DIRECTION ( 'NONE',  ( 0.8571428571428572063, -4.467596029561073242E-15, -0.5150787536377126052 ) ) ;
#22797=CARTESIAN_POINT ( 'NONE',  ( 7.980290731945706817, -0.6082991440336660283, 7.616182555102799512 ) ) ;
#22804=CARTESIAN_POINT ( 'NONE',  ( 12.84999999999997300, -12.00000000000011191, -6.249999999999936051 ) ) ;
#22806=CARTESIAN_POINT ( 'NONE',  ( -8.496394830447121294, -0.03251735406441521453, 6.998792816379902249 ) ) ;
#22811=CARTESIAN_POINT ( 'NONE',  ( -7.499999999999978684, -8.000000000000024869, 10.74999999999999645 ) ) ;
#22818=CIRCLE ( 'NONE', #1789, 0.4999999999999995559 ) ;
#22837=DIRECTION ( 'NONE',  ( -2.168404344970994323E-16, 1.000000000000000000, -1.577721810442023611E-30 ) ) ;
#22846=EDGE_CURVE ( 'NONE', #6039, #2116, #11915, .T. ) ;
#22847=AXIS2_PLACEMENT_3D ( 'NONE', #4626, #3347, #10386 ) ;
#22854=EDGE_LOOP ( 'NONE', ( #20484, #11210, #20191, #20076 ) ) ;
#22855=CARTESIAN_POINT ( 'NONE',  ( -12.85000000000001386, -12.00000000000008704, -2.549999999999958966 ) ) ;
#22860=CARTESIAN_POINT ( 'NONE',  ( -7.000000000000005329, -0.7870719649792564665, 9.239863038076329360 ) ) ;
#22861=CARTESIAN_POINT ( 'NONE',  ( -8.129778652391257410, -1.578738987863637089, 7.405931224841305394 ) ) ;
#22891=CARTESIAN_POINT ( 'NONE',  ( -7.980290731945705041, -13.39170085596635573, 7.616182555102821716 ) ) ;
#22901=FACE_BOUND ( 'NONE', #19003, .T. ) ;
#22910=ORIENTED_EDGE ( 'NONE', *, *, #5491, .F. ) ;
#22917=DIRECTION ( 'NONE',  ( -3.469446951953611428E-15, 1.000000000000000000, -3.469446951953610245E-15 ) ) ;
#22919=CARTESIAN_POINT ( 'NONE',  ( -8.697224362268011433, 6.938893903907228378E-15, 6.249999999999992006 ) ) ;
#22925=CARTESIAN_POINT ( 'NONE',  ( -8.115139842999401054, -0.1079360712687468249, 7.423524081915970463 ) ) ;
#22928=EDGE_CURVE ( 'NONE', #8955, #10857, #5947, .T. ) ;
#22931=CARTESIAN_POINT ( 'NONE',  ( -8.954763739086866181, -13.50000000000003553, 6.678571428571478563 ) ) ;
#22935=CARTESIAN_POINT ( 'NONE',  ( -12.84999999999999964, -2.000000000000001776, 2.549999999999997158 ) ) ;
#22948=DIRECTION ( 'NONE',  ( 0.5150787536377134934, 0.000000000000000000, 0.8571428571428567622 ) ) ;
#22973=LINE ( 'NONE', #6733, #22729 ) ;
#22974=CARTESIAN_POINT ( 'NONE',  ( 6.999999999999978684, -8.000000000000003553, 11.74999999999999645 ) ) ;
#22986=CARTESIAN_POINT ( 'NONE',  ( -7.595478965369722779, -11.97605770252013180, 8.489833260407468885 ) ) ;
#22999=VECTOR ( 'NONE', #13193, 1000.000000000000000 ) ;
#23008=CARTESIAN_POINT ( 'NONE',  ( -7.607945571813282903, -0.8975439866888990093, 8.443122311927307777 ) ) ;
#23013=AXIS2_PLACEMENT_3D ( 'NONE', #15900, #12610, #12843 ) ;
#23015=CARTESIAN_POINT ( 'NONE',  ( -7.955953741309929939, -1.644172503818049025, 7.654083333123823607 ) ) ;
#23023=AXIS2_PLACEMENT_3D ( 'NONE', #16408, #22071, #11345 ) ;
#23025=AXIS2_PLACEMENT_3D ( 'NONE', #11368, #11489, #13737 ) ;
#23052=CYLINDRICAL_SURFACE ( 'NONE', #21701, 2.999999999999995559 ) ;
#23067=CARTESIAN_POINT ( 'NONE',  ( -7.500000000000007105, -5.999999999999987566, 10.25000000000000888 ) ) ;
#23072=PLANE ( 'NONE',  #18544 ) ;
#23075=CARTESIAN_POINT ( 'NONE',  ( -12.85000000000004228, -1.499999999999997780, -6.249999999999977796 ) ) ;
#23076=CARTESIAN_POINT ( 'NONE',  ( -7.735962016526146456, -13.93008758169059824, 7.174192622767023408 ) ) ;
#23083=CARTESIAN_POINT ( 'NONE',  ( 12.84999999999999964, -12.50000000000011191, -6.249999999999921840 ) ) ;
#23090=ORIENTED_EDGE ( 'NONE', *, *, #8108, .F. ) ;
#23099=DIRECTION ( 'NONE',  ( 1.454462294001240516E-30, 1.000000000000000000, 7.888609052210128564E-31 ) ) ;
#23111=DIRECTION ( 'NONE',  ( -1.734723475976813750E-16, -1.000000000000000000, 3.469446951953607484E-15 ) ) ;
#23123=EDGE_LOOP ( 'NONE', ( #742, #4173, #4551, #17818 ) ) ;
#23124=VERTEX_POINT ( 'NONE', #6262 ) ;
#23132=FACE_OUTER_BOUND ( 'NONE', #11686, .T. ) ;
#23144=DIRECTION ( 'NONE',  ( 0.000000000000000000, -6.938893903907238633E-15, -1.000000000000000000 ) ) ;
#23150=AXIS2_PLACEMENT_3D ( 'NONE', #21676, #20014, #9310 ) ;
#23163=CARTESIAN_POINT ( 'NONE',  ( 7.499999999999978684, -8.000000000000051514, 6.249999999999977796 ) ) ;
#23170=AXIS2_PLACEMENT_3D ( 'NONE', #3731, #1398, #8573 ) ;
#23174=ORIENTED_EDGE ( 'NONE', *, *, #4481, .T. ) ;
#23180=ORIENTED_EDGE ( 'NONE', *, *, #7304, .F. ) ;
#23202=AXIS2_PLACEMENT_3D ( 'NONE', #20619, #8139, #2844 ) ;
#23213=FACE_BOUND ( 'NONE', #21957, .T. ) ;
#23216=CARTESIAN_POINT ( 'NONE',  ( 12.84999999999997300, -1.499999999999997780, 1.387778780781445676E-14 ) ) ;
#23223=DIRECTION ( 'NONE',  ( -0.8571428571428568732, 7.888609052210126812E-31, -0.5150787536377133824 ) ) ;
#23225=EDGE_CURVE ( 'NONE', #10857, #7917, #4242, .T. ) ;
#23247=VECTOR ( 'NONE', #19186, 1000.000000000000000 ) ;
#23250=CARTESIAN_POINT ( 'NONE',  ( -7.607945571813328201, -13.10245601331111587, 8.443122311927368173 ) ) ;
#23251=DIRECTION ( 'NONE',  ( 0.000000000000000000, 0.7453559924999302311, 0.6666666666666662966 ) ) ;
ENDSEC;
END-ISO-10303-21;
